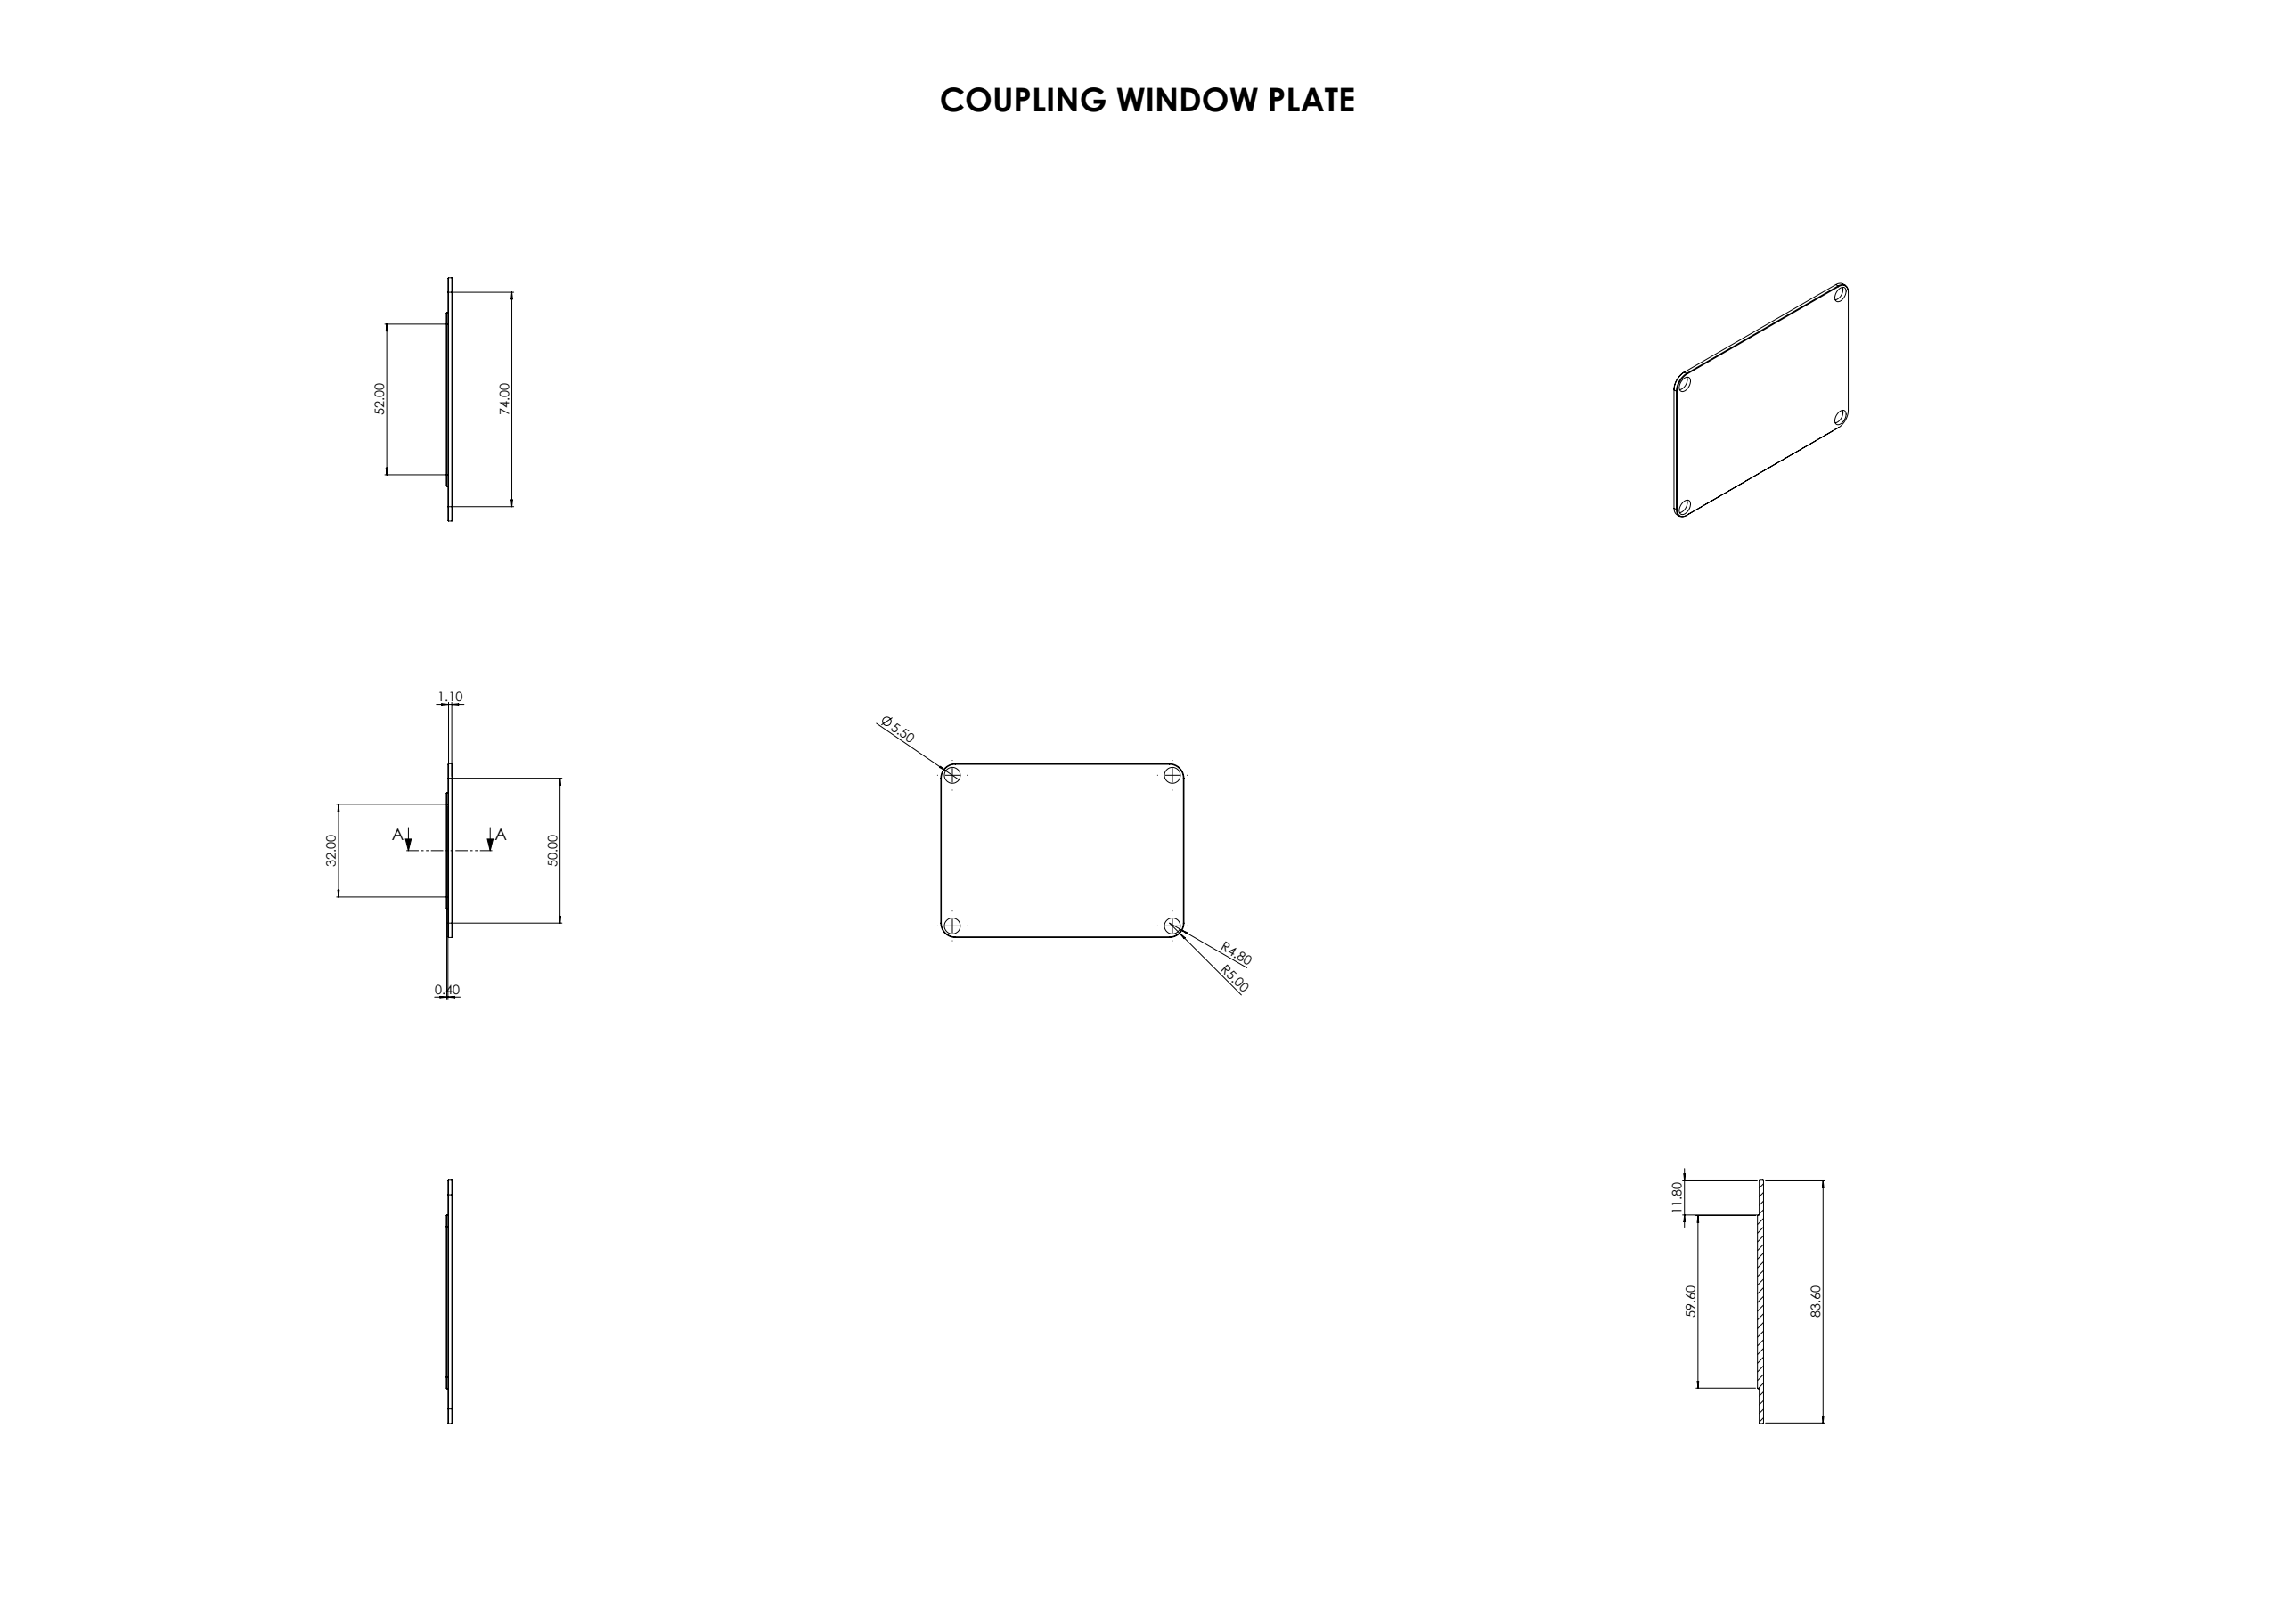
ISO-10303-21;
HEADER;
/* Generated by software containing ST-Developer
 * from STEP Tools, Inc. (www.steptools.com) 
 */

FILE_DESCRIPTION(
/* description */ (''),
/* implementation_level */ '2;1');

FILE_NAME(
/* name */ '18_Coupling_Window_Plate.step',
/* time_stamp */ '2026-10-26T04:15:57-07:00',
/* author */ (''),
/* organization */ (''),
/* preprocessor_version */ 'ST-DEVELOPER v20.2',
/* originating_system */ 'Autodesk Translation Framework v15.15.0.0',
/* authorisation */ '');

FILE_SCHEMA (('AUTOMOTIVE_DESIGN { 1 0 10303 214 3 1 1 }'));
ENDSEC;

DATA;
#10=MECHANICAL_DESIGN_GEOMETRIC_PRESENTATION_REPRESENTATION('',(#466),#55737);
#386=CONICAL_SURFACE('',#29308,4.90000000000002,0.785398163397446);
#387=CONICAL_SURFACE('',#29312,4.90000000000001,0.785398163397446);
#388=CONICAL_SURFACE('',#29316,4.90000000000003,0.785398163397493);
#389=CONICAL_SURFACE('',#29320,4.9,0.785398163397493);
#390=CONICAL_SURFACE('',#29339,4.9,0.785398163397493);
#391=CONICAL_SURFACE('',#29343,4.90000000000003,0.785398163397493);
#392=CONICAL_SURFACE('',#29347,4.90000000000001,0.785398163397446);
#393=CONICAL_SURFACE('',#29350,4.90000000000002,0.785398163397446);
#394=CONICAL_SURFACE('',#29361,3.90000000000002,0.785398163397454);
#395=CONICAL_SURFACE('',#29365,3.90000000000002,0.785398163397446);
#396=CONICAL_SURFACE('',#29369,3.89999999999998,0.785398163397493);
#397=CONICAL_SURFACE('',#29373,3.89999999999997,0.785398163397493);
#426=SHAPE_REPRESENTATION_RELATIONSHIP('SRR','None',#55835,#446);
#446=ADVANCED_BREP_SHAPE_REPRESENTATION('',(#486),#55731);
#466=STYLED_ITEM('',(#55977),#486);
#486=MANIFOLD_SOLID_BREP('Body1',#27235);
#704=FACE_BOUND('',#9610,.T.);
#705=FACE_BOUND('',#9611,.T.);
#706=FACE_BOUND('',#9612,.T.);
#707=FACE_BOUND('',#9613,.T.);
#708=FACE_BOUND('',#9614,.T.);
#709=FACE_BOUND('',#9627,.T.);
#710=FACE_BOUND('',#9628,.T.);
#711=FACE_BOUND('',#9629,.T.);
#712=FACE_BOUND('',#9630,.T.);
#1451=PLANE('',#29307);
#1452=PLANE('',#29311);
#1453=PLANE('',#29315);
#1454=PLANE('',#29319);
#1455=PLANE('',#29325);
#1456=PLANE('',#29328);
#1457=PLANE('',#29329);
#1458=PLANE('',#29338);
#1459=PLANE('',#29342);
#1460=PLANE('',#29346);
#1461=PLANE('',#29349);
#1462=PLANE('',#29353);
#1463=PLANE('',#29355);
#1464=PLANE('',#29360);
#1465=PLANE('',#29364);
#1466=PLANE('',#29368);
#1467=PLANE('',#29372);
#1468=PLANE('',#29377);
#1469=PLANE('',#29379);
#1470=PLANE('',#29380);
#1471=PLANE('',#29382);
#1472=PLANE('',#29384);
#1473=PLANE('',#29389);
#3420=LINE('',#45873,#5791);
#3421=LINE('',#45875,#5792);
#3422=LINE('',#45877,#5793);
#3423=LINE('',#45878,#5794);
#3424=LINE('',#45882,#5795);
#3425=LINE('',#45888,#5796);
#3426=LINE('',#45889,#5797);
#3427=LINE('',#45890,#5798);
#3428=LINE('',#45894,#5799);
#3429=LINE('',#45900,#5800);
#3430=LINE('',#45901,#5801);
#3431=LINE('',#45902,#5802);
#3432=LINE('',#45906,#5803);
#3433=LINE('',#45912,#5804);
#3434=LINE('',#45913,#5805);
#3435=LINE('',#45914,#5806);
#3436=LINE('',#45920,#5807);
#3437=LINE('',#45923,#5808);
#3438=LINE('',#45926,#5809);
#3439=LINE('',#45927,#5810);
#3440=LINE('',#45930,#5811);
#3441=LINE('',#45934,#5812);
#3442=LINE('',#45935,#5813);
#3443=LINE('',#45947,#5814);
#3444=LINE('',#45951,#5815);
#3445=LINE('',#45955,#5816);
#3446=LINE('',#45959,#5817);
#3447=LINE('',#45963,#5818);
#3448=LINE('',#45965,#5819);
#3449=LINE('',#45966,#5820);
#3450=LINE('',#45970,#5821);
#3451=LINE('',#45976,#5822);
#3452=LINE('',#45977,#5823);
#3453=LINE('',#45978,#5824);
#3454=LINE('',#45982,#5825);
#3455=LINE('',#45987,#5826);
#3456=LINE('',#45988,#5827);
#3457=LINE('',#45989,#5828);
#3458=LINE('',#45992,#5829);
#3459=LINE('',#45996,#5830);
#3460=LINE('',#45997,#5831);
#3461=LINE('',#46001,#5832);
#3462=LINE('',#46002,#5833);
#3463=LINE('',#46004,#5834);
#3464=LINE('',#46018,#5835);
#3465=LINE('',#46020,#5836);
#3466=LINE('',#46022,#5837);
#3467=LINE('',#46023,#5838);
#3468=LINE('',#46027,#5839);
#3469=LINE('',#46033,#5840);
#3470=LINE('',#46034,#5841);
#3471=LINE('',#46035,#5842);
#3472=LINE('',#46039,#5843);
#3473=LINE('',#46045,#5844);
#3474=LINE('',#46046,#5845);
#3475=LINE('',#46047,#5846);
#3476=LINE('',#46051,#5847);
#3477=LINE('',#46057,#5848);
#3478=LINE('',#46058,#5849);
#3479=LINE('',#46059,#5850);
#3480=LINE('',#46064,#5851);
#3481=LINE('',#46065,#5852);
#3482=LINE('',#46067,#5853);
#3483=LINE('',#46069,#5854);
#3484=LINE('',#46071,#5855);
#3485=LINE('',#46074,#5856);
#3486=LINE('',#46076,#5857);
#3487=LINE('',#46078,#5858);
#3488=LINE('',#46081,#5859);
#3489=LINE('',#46083,#5860);
#3490=LINE('',#46085,#5861);
#3491=LINE('',#46087,#5862);
#5791=VECTOR('',#35330,10.);
#5792=VECTOR('',#35331,10.);
#5793=VECTOR('',#35332,10.);
#5794=VECTOR('',#35333,10.);
#5795=VECTOR('',#35336,10.);
#5796=VECTOR('',#35343,10.);
#5797=VECTOR('',#35344,10.);
#5798=VECTOR('',#35345,10.);
#5799=VECTOR('',#35348,10.);
#5800=VECTOR('',#35355,10.);
#5801=VECTOR('',#35356,10.);
#5802=VECTOR('',#35357,10.);
#5803=VECTOR('',#35360,10.);
#5804=VECTOR('',#35367,10.);
#5805=VECTOR('',#35368,10.);
#5806=VECTOR('',#35369,10.);
#5807=VECTOR('',#35378,10.);
#5808=VECTOR('',#35381,10.);
#5809=VECTOR('',#35384,10.);
#5810=VECTOR('',#35385,10.);
#5811=VECTOR('',#35388,10.);
#5812=VECTOR('',#35393,10.);
#5813=VECTOR('',#35394,10.);
#5814=VECTOR('',#35405,10.);
#5815=VECTOR('',#35408,10.);
#5816=VECTOR('',#35411,10.);
#5817=VECTOR('',#35414,10.);
#5818=VECTOR('',#35419,10.);
#5819=VECTOR('',#35420,10.);
#5820=VECTOR('',#35421,10.);
#5821=VECTOR('',#35424,10.);
#5822=VECTOR('',#35431,10.);
#5823=VECTOR('',#35432,10.);
#5824=VECTOR('',#35433,10.);
#5825=VECTOR('',#35436,10.);
#5826=VECTOR('',#35443,10.);
#5827=VECTOR('',#35444,10.);
#5828=VECTOR('',#35445,10.);
#5829=VECTOR('',#35448,10.);
#5830=VECTOR('',#35453,10.);
#5831=VECTOR('',#35454,10.);
#5832=VECTOR('',#35461,10.);
#5833=VECTOR('',#35462,10.);
#5834=VECTOR('',#35465,10.);
#5835=VECTOR('',#35480,10.);
#5836=VECTOR('',#35481,10.);
#5837=VECTOR('',#35482,10.);
#5838=VECTOR('',#35483,10.);
#5839=VECTOR('',#35486,10.);
#5840=VECTOR('',#35493,10.);
#5841=VECTOR('',#35494,10.);
#5842=VECTOR('',#35495,10.);
#5843=VECTOR('',#35498,10.);
#5844=VECTOR('',#35505,10.);
#5845=VECTOR('',#35506,10.);
#5846=VECTOR('',#35507,10.);
#5847=VECTOR('',#35510,10.);
#5848=VECTOR('',#35517,10.);
#5849=VECTOR('',#35518,10.);
#5850=VECTOR('',#35519,10.);
#5851=VECTOR('',#35528,10.);
#5852=VECTOR('',#35529,10.);
#5853=VECTOR('',#35532,10.);
#5854=VECTOR('',#35535,10.);
#5855=VECTOR('',#35538,10.);
#5856=VECTOR('',#35543,10.);
#5857=VECTOR('',#35546,10.);
#5858=VECTOR('',#35549,10.);
#5859=VECTOR('',#35554,2.75);
#5860=VECTOR('',#35557,2.75);
#5861=VECTOR('',#35560,2.75);
#5862=VECTOR('',#35563,2.75);
#6699=CYLINDRICAL_SURFACE('',#29323,5.00000000000001);
#6700=CYLINDRICAL_SURFACE('',#29326,5.00000000000002);
#6701=CYLINDRICAL_SURFACE('',#29352,5.00000000000004);
#6702=CYLINDRICAL_SURFACE('',#29354,5.00000000000001);
#6703=CYLINDRICAL_SURFACE('',#29376,4.00000000000002);
#6704=CYLINDRICAL_SURFACE('',#29378,4.00000000000002);
#6705=CYLINDRICAL_SURFACE('',#29381,3.99999999999998);
#6706=CYLINDRICAL_SURFACE('',#29383,3.99999999999999);
#6707=CYLINDRICAL_SURFACE('',#29385,2.75);
#6708=CYLINDRICAL_SURFACE('',#29386,2.75);
#6709=CYLINDRICAL_SURFACE('',#29387,2.75);
#6710=CYLINDRICAL_SURFACE('',#29388,2.75);
#7928=FACE_OUTER_BOUND('',#9597,.T.);
#7929=FACE_OUTER_BOUND('',#9598,.T.);
#7930=FACE_OUTER_BOUND('',#9599,.T.);
#7931=FACE_OUTER_BOUND('',#9600,.T.);
#7932=FACE_OUTER_BOUND('',#9601,.T.);
#7933=FACE_OUTER_BOUND('',#9602,.T.);
#7934=FACE_OUTER_BOUND('',#9603,.T.);
#7935=FACE_OUTER_BOUND('',#9604,.T.);
#7936=FACE_OUTER_BOUND('',#9605,.T.);
#7937=FACE_OUTER_BOUND('',#9606,.T.);
#7938=FACE_OUTER_BOUND('',#9607,.T.);
#7939=FACE_OUTER_BOUND('',#9608,.T.);
#7940=FACE_OUTER_BOUND('',#9609,.T.);
#7941=FACE_OUTER_BOUND('',#9615,.T.);
#7942=FACE_OUTER_BOUND('',#9616,.T.);
#7943=FACE_OUTER_BOUND('',#9617,.T.);
#7944=FACE_OUTER_BOUND('',#9618,.T.);
#7945=FACE_OUTER_BOUND('',#9619,.T.);
#7946=FACE_OUTER_BOUND('',#9620,.T.);
#7947=FACE_OUTER_BOUND('',#9621,.T.);
#7948=FACE_OUTER_BOUND('',#9622,.T.);
#7949=FACE_OUTER_BOUND('',#9623,.T.);
#7950=FACE_OUTER_BOUND('',#9624,.T.);
#7951=FACE_OUTER_BOUND('',#9625,.T.);
#7952=FACE_OUTER_BOUND('',#9626,.T.);
#7953=FACE_OUTER_BOUND('',#9631,.T.);
#7954=FACE_OUTER_BOUND('',#9632,.T.);
#7955=FACE_OUTER_BOUND('',#9633,.T.);
#7956=FACE_OUTER_BOUND('',#9634,.T.);
#7957=FACE_OUTER_BOUND('',#9635,.T.);
#7958=FACE_OUTER_BOUND('',#9636,.T.);
#7959=FACE_OUTER_BOUND('',#9637,.T.);
#7960=FACE_OUTER_BOUND('',#9638,.T.);
#7961=FACE_OUTER_BOUND('',#9639,.T.);
#7962=FACE_OUTER_BOUND('',#9640,.T.);
#7963=FACE_OUTER_BOUND('',#9641,.T.);
#7964=FACE_OUTER_BOUND('',#9642,.T.);
#7965=FACE_OUTER_BOUND('',#9643,.T.);
#7966=FACE_OUTER_BOUND('',#9644,.T.);
#7967=FACE_OUTER_BOUND('',#9645,.T.);
#7968=FACE_OUTER_BOUND('',#9646,.T.);
#7969=FACE_OUTER_BOUND('',#9647,.T.);
#7970=FACE_OUTER_BOUND('',#9648,.T.);
#7971=FACE_OUTER_BOUND('',#9649,.T.);
#7972=FACE_OUTER_BOUND('',#9650,.T.);
#7973=FACE_OUTER_BOUND('',#9651,.T.);
#7974=FACE_OUTER_BOUND('',#9652,.T.);
#9597=EDGE_LOOP('',(#23306,#23307,#23308,#23309));
#9598=EDGE_LOOP('',(#23310,#23311,#23312,#23313));
#9599=EDGE_LOOP('',(#23314,#23315,#23316,#23317));
#9600=EDGE_LOOP('',(#23318,#23319,#23320,#23321));
#9601=EDGE_LOOP('',(#23322,#23323,#23324,#23325));
#9602=EDGE_LOOP('',(#23326,#23327,#23328,#23329));
#9603=EDGE_LOOP('',(#23330,#23331,#23332,#23333));
#9604=EDGE_LOOP('',(#23334,#23335,#23336,#23337));
#9605=EDGE_LOOP('',(#23338,#23339,#23340,#23341));
#9606=EDGE_LOOP('',(#23342,#23343,#23344,#23345));
#9607=EDGE_LOOP('',(#23346,#23347,#23348,#23349));
#9608=EDGE_LOOP('',(#23350,#23351,#23352,#23353));
#9609=EDGE_LOOP('',(#23354,#23355,#23356,#23357,#23358,#23359,#23360,#23361));
#9610=EDGE_LOOP('',(#23362));
#9611=EDGE_LOOP('',(#23363));
#9612=EDGE_LOOP('',(#23364));
#9613=EDGE_LOOP('',(#23365));
#9614=EDGE_LOOP('',(#23366,#23367,#23368,#23369,#23370,#23371,#23372,#23373));
#9615=EDGE_LOOP('',(#23374,#23375,#23376,#23377));
#9616=EDGE_LOOP('',(#23378,#23379,#23380,#23381));
#9617=EDGE_LOOP('',(#23382,#23383,#23384,#23385));
#9618=EDGE_LOOP('',(#23386,#23387,#23388,#23389));
#9619=EDGE_LOOP('',(#23390,#23391,#23392,#23393));
#9620=EDGE_LOOP('',(#23394,#23395,#23396,#23397));
#9621=EDGE_LOOP('',(#23398,#23399,#23400,#23401));
#9622=EDGE_LOOP('',(#23402,#23403,#23404,#23405));
#9623=EDGE_LOOP('',(#23406,#23407,#23408,#23409));
#9624=EDGE_LOOP('',(#23410,#23411,#23412,#23413));
#9625=EDGE_LOOP('',(#23414,#23415,#23416,#23417));
#9626=EDGE_LOOP('',(#23418,#23419,#23420,#23421,#23422,#23423,#23424,#23425));
#9627=EDGE_LOOP('',(#23426));
#9628=EDGE_LOOP('',(#23427));
#9629=EDGE_LOOP('',(#23428));
#9630=EDGE_LOOP('',(#23429));
#9631=EDGE_LOOP('',(#23430,#23431,#23432,#23433));
#9632=EDGE_LOOP('',(#23434,#23435,#23436,#23437));
#9633=EDGE_LOOP('',(#23438,#23439,#23440,#23441));
#9634=EDGE_LOOP('',(#23442,#23443,#23444,#23445));
#9635=EDGE_LOOP('',(#23446,#23447,#23448,#23449));
#9636=EDGE_LOOP('',(#23450,#23451,#23452,#23453));
#9637=EDGE_LOOP('',(#23454,#23455,#23456,#23457));
#9638=EDGE_LOOP('',(#23458,#23459,#23460,#23461));
#9639=EDGE_LOOP('',(#23462,#23463,#23464,#23465));
#9640=EDGE_LOOP('',(#23466,#23467,#23468,#23469));
#9641=EDGE_LOOP('',(#23470,#23471,#23472,#23473));
#9642=EDGE_LOOP('',(#23474,#23475,#23476,#23477));
#9643=EDGE_LOOP('',(#23478,#23479,#23480,#23481,#23482,#23483,#23484,#23485));
#9644=EDGE_LOOP('',(#23486,#23487,#23488,#23489));
#9645=EDGE_LOOP('',(#23490,#23491,#23492,#23493));
#9646=EDGE_LOOP('',(#23494,#23495,#23496,#23497));
#9647=EDGE_LOOP('',(#23498,#23499,#23500,#23501));
#9648=EDGE_LOOP('',(#23502,#23503,#23504,#23505));
#9649=EDGE_LOOP('',(#23506,#23507,#23508,#23509));
#9650=EDGE_LOOP('',(#23510,#23511,#23512,#23513));
#9651=EDGE_LOOP('',(#23514,#23515,#23516,#23517));
#9652=EDGE_LOOP('',(#23518,#23519,#23520,#23521));
#10811=CIRCLE('',#29309,4.80000000000002);
#10812=CIRCLE('',#29310,5.00000000000002);
#10813=CIRCLE('',#29313,4.80000000000001);
#10814=CIRCLE('',#29314,5.00000000000001);
#10815=CIRCLE('',#29317,4.80000000000002);
#10816=CIRCLE('',#29318,5.00000000000004);
#10817=CIRCLE('',#29321,4.8);
#10818=CIRCLE('',#29322,5.00000000000001);
#10819=CIRCLE('',#29324,5.00000000000001);
#10820=CIRCLE('',#29327,5.00000000000002);
#10821=CIRCLE('',#29330,2.75);
#10822=CIRCLE('',#29331,2.75);
#10823=CIRCLE('',#29332,2.75);
#10824=CIRCLE('',#29333,2.75);
#10825=CIRCLE('',#29334,3.99999999999998);
#10826=CIRCLE('',#29335,3.99999999999999);
#10827=CIRCLE('',#29336,4.00000000000002);
#10828=CIRCLE('',#29337,4.00000000000002);
#10829=CIRCLE('',#29340,4.8);
#10830=CIRCLE('',#29341,5.00000000000001);
#10831=CIRCLE('',#29344,4.80000000000002);
#10832=CIRCLE('',#29345,5.00000000000004);
#10833=CIRCLE('',#29348,4.80000000000001);
#10834=CIRCLE('',#29351,4.80000000000002);
#10835=CIRCLE('',#29356,2.75);
#10836=CIRCLE('',#29357,2.75);
#10837=CIRCLE('',#29358,2.75);
#10838=CIRCLE('',#29359,2.75);
#10839=CIRCLE('',#29362,3.80000000000002);
#10840=CIRCLE('',#29363,4.00000000000002);
#10841=CIRCLE('',#29366,3.80000000000002);
#10842=CIRCLE('',#29367,4.00000000000002);
#10843=CIRCLE('',#29370,3.79999999999997);
#10844=CIRCLE('',#29371,3.99999999999999);
#10845=CIRCLE('',#29374,3.79999999999997);
#10846=CIRCLE('',#29375,3.99999999999998);
#13176=VERTEX_POINT('',#45871);
#13177=VERTEX_POINT('',#45872);
#13178=VERTEX_POINT('',#45874);
#13179=VERTEX_POINT('',#45876);
#13180=VERTEX_POINT('',#45880);
#13181=VERTEX_POINT('',#45881);
#13182=VERTEX_POINT('',#45886);
#13183=VERTEX_POINT('',#45887);
#13184=VERTEX_POINT('',#45892);
#13185=VERTEX_POINT('',#45893);
#13186=VERTEX_POINT('',#45898);
#13187=VERTEX_POINT('',#45899);
#13188=VERTEX_POINT('',#45904);
#13189=VERTEX_POINT('',#45905);
#13190=VERTEX_POINT('',#45910);
#13191=VERTEX_POINT('',#45911);
#13192=VERTEX_POINT('',#45919);
#13193=VERTEX_POINT('',#45921);
#13194=VERTEX_POINT('',#45925);
#13195=VERTEX_POINT('',#45929);
#13196=VERTEX_POINT('',#45933);
#13197=VERTEX_POINT('',#45937);
#13198=VERTEX_POINT('',#45939);
#13199=VERTEX_POINT('',#45941);
#13200=VERTEX_POINT('',#45943);
#13201=VERTEX_POINT('',#45945);
#13202=VERTEX_POINT('',#45946);
#13203=VERTEX_POINT('',#45948);
#13204=VERTEX_POINT('',#45950);
#13205=VERTEX_POINT('',#45952);
#13206=VERTEX_POINT('',#45954);
#13207=VERTEX_POINT('',#45956);
#13208=VERTEX_POINT('',#45958);
#13209=VERTEX_POINT('',#45962);
#13210=VERTEX_POINT('',#45964);
#13211=VERTEX_POINT('',#45968);
#13212=VERTEX_POINT('',#45969);
#13213=VERTEX_POINT('',#45974);
#13214=VERTEX_POINT('',#45975);
#13215=VERTEX_POINT('',#45980);
#13216=VERTEX_POINT('',#45981);
#13217=VERTEX_POINT('',#45986);
#13218=VERTEX_POINT('',#45991);
#13219=VERTEX_POINT('',#45995);
#13220=VERTEX_POINT('',#46007);
#13221=VERTEX_POINT('',#46009);
#13222=VERTEX_POINT('',#46011);
#13223=VERTEX_POINT('',#46013);
#13224=VERTEX_POINT('',#46016);
#13225=VERTEX_POINT('',#46017);
#13226=VERTEX_POINT('',#46019);
#13227=VERTEX_POINT('',#46021);
#13228=VERTEX_POINT('',#46025);
#13229=VERTEX_POINT('',#46026);
#13230=VERTEX_POINT('',#46031);
#13231=VERTEX_POINT('',#46032);
#13232=VERTEX_POINT('',#46037);
#13233=VERTEX_POINT('',#46038);
#13234=VERTEX_POINT('',#46043);
#13235=VERTEX_POINT('',#46044);
#13236=VERTEX_POINT('',#46049);
#13237=VERTEX_POINT('',#46050);
#13238=VERTEX_POINT('',#46055);
#13239=VERTEX_POINT('',#46056);
#16657=EDGE_CURVE('',#13176,#13177,#3420,.T.);
#16658=EDGE_CURVE('',#13177,#13178,#3421,.T.);
#16659=EDGE_CURVE('',#13178,#13179,#3422,.T.);
#16660=EDGE_CURVE('',#13179,#13176,#3423,.T.);
#16661=EDGE_CURVE('',#13180,#13181,#3424,.T.);
#16662=EDGE_CURVE('',#13181,#13177,#10811,.T.);
#16663=EDGE_CURVE('',#13176,#13180,#10812,.T.);
#16664=EDGE_CURVE('',#13182,#13183,#3425,.T.);
#16665=EDGE_CURVE('',#13183,#13181,#3426,.T.);
#16666=EDGE_CURVE('',#13180,#13182,#3427,.T.);
#16667=EDGE_CURVE('',#13184,#13185,#3428,.T.);
#16668=EDGE_CURVE('',#13185,#13183,#10813,.T.);
#16669=EDGE_CURVE('',#13182,#13184,#10814,.T.);
#16670=EDGE_CURVE('',#13186,#13187,#3429,.T.);
#16671=EDGE_CURVE('',#13187,#13185,#3430,.T.);
#16672=EDGE_CURVE('',#13184,#13186,#3431,.T.);
#16673=EDGE_CURVE('',#13188,#13189,#3432,.T.);
#16674=EDGE_CURVE('',#13189,#13187,#10815,.T.);
#16675=EDGE_CURVE('',#13186,#13188,#10816,.T.);
#16676=EDGE_CURVE('',#13190,#13191,#3433,.T.);
#16677=EDGE_CURVE('',#13191,#13189,#3434,.T.);
#16678=EDGE_CURVE('',#13188,#13190,#3435,.T.);
#16679=EDGE_CURVE('',#13178,#13191,#10817,.T.);
#16680=EDGE_CURVE('',#13190,#13179,#10818,.T.);
#16681=EDGE_CURVE('',#13192,#13182,#3436,.T.);
#16682=EDGE_CURVE('',#13193,#13192,#10819,.T.);
#16683=EDGE_CURVE('',#13193,#13184,#3437,.T.);
#16684=EDGE_CURVE('',#13194,#13180,#3438,.T.);
#16685=EDGE_CURVE('',#13192,#13194,#3439,.T.);
#16686=EDGE_CURVE('',#13195,#13176,#3440,.T.);
#16687=EDGE_CURVE('',#13194,#13195,#10820,.T.);
#16688=EDGE_CURVE('',#13196,#13179,#3441,.T.);
#16689=EDGE_CURVE('',#13195,#13196,#3442,.T.);
#16690=EDGE_CURVE('',#13197,#13197,#10821,.T.);
#16691=EDGE_CURVE('',#13198,#13198,#10822,.T.);
#16692=EDGE_CURVE('',#13199,#13199,#10823,.T.);
#16693=EDGE_CURVE('',#13200,#13200,#10824,.T.);
#16694=EDGE_CURVE('',#13201,#13202,#3443,.T.);
#16695=EDGE_CURVE('',#13202,#13203,#10825,.T.);
#16696=EDGE_CURVE('',#13203,#13204,#3444,.T.);
#16697=EDGE_CURVE('',#13204,#13205,#10826,.T.);
#16698=EDGE_CURVE('',#13205,#13206,#3445,.T.);
#16699=EDGE_CURVE('',#13206,#13207,#10827,.T.);
#16700=EDGE_CURVE('',#13207,#13208,#3446,.T.);
#16701=EDGE_CURVE('',#13208,#13201,#10828,.T.);
#16702=EDGE_CURVE('',#13196,#13209,#3447,.T.);
#16703=EDGE_CURVE('',#13209,#13210,#3448,.T.);
#16704=EDGE_CURVE('',#13210,#13195,#3449,.T.);
#16705=EDGE_CURVE('',#13211,#13212,#3450,.T.);
#16706=EDGE_CURVE('',#13212,#13209,#10829,.T.);
#16707=EDGE_CURVE('',#13196,#13211,#10830,.T.);
#16708=EDGE_CURVE('',#13213,#13214,#3451,.T.);
#16709=EDGE_CURVE('',#13214,#13212,#3452,.T.);
#16710=EDGE_CURVE('',#13211,#13213,#3453,.T.);
#16711=EDGE_CURVE('',#13215,#13216,#3454,.T.);
#16712=EDGE_CURVE('',#13216,#13214,#10831,.T.);
#16713=EDGE_CURVE('',#13213,#13215,#10832,.T.);
#16714=EDGE_CURVE('',#13193,#13217,#3455,.T.);
#16715=EDGE_CURVE('',#13217,#13216,#3456,.T.);
#16716=EDGE_CURVE('',#13215,#13193,#3457,.T.);
#16717=EDGE_CURVE('',#13192,#13218,#3458,.T.);
#16718=EDGE_CURVE('',#13218,#13217,#10833,.T.);
#16719=EDGE_CURVE('',#13194,#13219,#3459,.T.);
#16720=EDGE_CURVE('',#13219,#13218,#3460,.T.);
#16721=EDGE_CURVE('',#13210,#13219,#10834,.T.);
#16722=EDGE_CURVE('',#13215,#13186,#3461,.T.);
#16723=EDGE_CURVE('',#13213,#13188,#3462,.T.);
#16724=EDGE_CURVE('',#13211,#13190,#3463,.T.);
#16725=EDGE_CURVE('',#13220,#13220,#10835,.T.);
#16726=EDGE_CURVE('',#13221,#13221,#10836,.T.);
#16727=EDGE_CURVE('',#13222,#13222,#10837,.T.);
#16728=EDGE_CURVE('',#13223,#13223,#10838,.T.);
#16729=EDGE_CURVE('',#13224,#13225,#3464,.T.);
#16730=EDGE_CURVE('',#13225,#13226,#3465,.T.);
#16731=EDGE_CURVE('',#13226,#13227,#3466,.T.);
#16732=EDGE_CURVE('',#13227,#13224,#3467,.T.);
#16733=EDGE_CURVE('',#13228,#13229,#3468,.T.);
#16734=EDGE_CURVE('',#13229,#13225,#10839,.T.);
#16735=EDGE_CURVE('',#13224,#13228,#10840,.T.);
#16736=EDGE_CURVE('',#13230,#13231,#3469,.T.);
#16737=EDGE_CURVE('',#13231,#13229,#3470,.T.);
#16738=EDGE_CURVE('',#13228,#13230,#3471,.T.);
#16739=EDGE_CURVE('',#13232,#13233,#3472,.T.);
#16740=EDGE_CURVE('',#13233,#13231,#10841,.T.);
#16741=EDGE_CURVE('',#13230,#13232,#10842,.T.);
#16742=EDGE_CURVE('',#13234,#13235,#3473,.T.);
#16743=EDGE_CURVE('',#13235,#13233,#3474,.T.);
#16744=EDGE_CURVE('',#13232,#13234,#3475,.T.);
#16745=EDGE_CURVE('',#13236,#13237,#3476,.T.);
#16746=EDGE_CURVE('',#13237,#13235,#10843,.T.);
#16747=EDGE_CURVE('',#13234,#13236,#10844,.T.);
#16748=EDGE_CURVE('',#13238,#13239,#3477,.T.);
#16749=EDGE_CURVE('',#13239,#13237,#3478,.T.);
#16750=EDGE_CURVE('',#13236,#13238,#3479,.T.);
#16751=EDGE_CURVE('',#13226,#13239,#10845,.T.);
#16752=EDGE_CURVE('',#13238,#13227,#10846,.T.);
#16753=EDGE_CURVE('',#13207,#13230,#3480,.T.);
#16754=EDGE_CURVE('',#13206,#13232,#3481,.T.);
#16755=EDGE_CURVE('',#13208,#13228,#3482,.T.);
#16756=EDGE_CURVE('',#13201,#13224,#3483,.T.);
#16757=EDGE_CURVE('',#13202,#13227,#3484,.T.);
#16758=EDGE_CURVE('',#13203,#13238,#3485,.T.);
#16759=EDGE_CURVE('',#13204,#13236,#3486,.T.);
#16760=EDGE_CURVE('',#13205,#13234,#3487,.T.);
#16761=EDGE_CURVE('',#13223,#13200,#3488,.T.);
#16762=EDGE_CURVE('',#13222,#13199,#3489,.T.);
#16763=EDGE_CURVE('',#13221,#13198,#3490,.T.);
#16764=EDGE_CURVE('',#13220,#13197,#3491,.T.);
#23306=ORIENTED_EDGE('',*,*,#16657,.T.);
#23307=ORIENTED_EDGE('',*,*,#16658,.T.);
#23308=ORIENTED_EDGE('',*,*,#16659,.T.);
#23309=ORIENTED_EDGE('',*,*,#16660,.T.);
#23310=ORIENTED_EDGE('',*,*,#16661,.T.);
#23311=ORIENTED_EDGE('',*,*,#16662,.T.);
#23312=ORIENTED_EDGE('',*,*,#16657,.F.);
#23313=ORIENTED_EDGE('',*,*,#16663,.T.);
#23314=ORIENTED_EDGE('',*,*,#16664,.T.);
#23315=ORIENTED_EDGE('',*,*,#16665,.T.);
#23316=ORIENTED_EDGE('',*,*,#16661,.F.);
#23317=ORIENTED_EDGE('',*,*,#16666,.T.);
#23318=ORIENTED_EDGE('',*,*,#16667,.T.);
#23319=ORIENTED_EDGE('',*,*,#16668,.T.);
#23320=ORIENTED_EDGE('',*,*,#16664,.F.);
#23321=ORIENTED_EDGE('',*,*,#16669,.T.);
#23322=ORIENTED_EDGE('',*,*,#16670,.T.);
#23323=ORIENTED_EDGE('',*,*,#16671,.T.);
#23324=ORIENTED_EDGE('',*,*,#16667,.F.);
#23325=ORIENTED_EDGE('',*,*,#16672,.T.);
#23326=ORIENTED_EDGE('',*,*,#16673,.T.);
#23327=ORIENTED_EDGE('',*,*,#16674,.T.);
#23328=ORIENTED_EDGE('',*,*,#16670,.F.);
#23329=ORIENTED_EDGE('',*,*,#16675,.T.);
#23330=ORIENTED_EDGE('',*,*,#16676,.T.);
#23331=ORIENTED_EDGE('',*,*,#16677,.T.);
#23332=ORIENTED_EDGE('',*,*,#16673,.F.);
#23333=ORIENTED_EDGE('',*,*,#16678,.T.);
#23334=ORIENTED_EDGE('',*,*,#16659,.F.);
#23335=ORIENTED_EDGE('',*,*,#16679,.T.);
#23336=ORIENTED_EDGE('',*,*,#16676,.F.);
#23337=ORIENTED_EDGE('',*,*,#16680,.T.);
#23338=ORIENTED_EDGE('',*,*,#16669,.F.);
#23339=ORIENTED_EDGE('',*,*,#16681,.F.);
#23340=ORIENTED_EDGE('',*,*,#16682,.F.);
#23341=ORIENTED_EDGE('',*,*,#16683,.T.);
#23342=ORIENTED_EDGE('',*,*,#16666,.F.);
#23343=ORIENTED_EDGE('',*,*,#16684,.F.);
#23344=ORIENTED_EDGE('',*,*,#16685,.F.);
#23345=ORIENTED_EDGE('',*,*,#16681,.T.);
#23346=ORIENTED_EDGE('',*,*,#16663,.F.);
#23347=ORIENTED_EDGE('',*,*,#16686,.F.);
#23348=ORIENTED_EDGE('',*,*,#16687,.F.);
#23349=ORIENTED_EDGE('',*,*,#16684,.T.);
#23350=ORIENTED_EDGE('',*,*,#16660,.F.);
#23351=ORIENTED_EDGE('',*,*,#16688,.F.);
#23352=ORIENTED_EDGE('',*,*,#16689,.F.);
#23353=ORIENTED_EDGE('',*,*,#16686,.T.);
#23354=ORIENTED_EDGE('',*,*,#16658,.F.);
#23355=ORIENTED_EDGE('',*,*,#16662,.F.);
#23356=ORIENTED_EDGE('',*,*,#16665,.F.);
#23357=ORIENTED_EDGE('',*,*,#16668,.F.);
#23358=ORIENTED_EDGE('',*,*,#16671,.F.);
#23359=ORIENTED_EDGE('',*,*,#16674,.F.);
#23360=ORIENTED_EDGE('',*,*,#16677,.F.);
#23361=ORIENTED_EDGE('',*,*,#16679,.F.);
#23362=ORIENTED_EDGE('',*,*,#16690,.T.);
#23363=ORIENTED_EDGE('',*,*,#16691,.T.);
#23364=ORIENTED_EDGE('',*,*,#16692,.T.);
#23365=ORIENTED_EDGE('',*,*,#16693,.T.);
#23366=ORIENTED_EDGE('',*,*,#16694,.T.);
#23367=ORIENTED_EDGE('',*,*,#16695,.T.);
#23368=ORIENTED_EDGE('',*,*,#16696,.T.);
#23369=ORIENTED_EDGE('',*,*,#16697,.T.);
#23370=ORIENTED_EDGE('',*,*,#16698,.T.);
#23371=ORIENTED_EDGE('',*,*,#16699,.T.);
#23372=ORIENTED_EDGE('',*,*,#16700,.T.);
#23373=ORIENTED_EDGE('',*,*,#16701,.T.);
#23374=ORIENTED_EDGE('',*,*,#16702,.T.);
#23375=ORIENTED_EDGE('',*,*,#16703,.T.);
#23376=ORIENTED_EDGE('',*,*,#16704,.T.);
#23377=ORIENTED_EDGE('',*,*,#16689,.T.);
#23378=ORIENTED_EDGE('',*,*,#16705,.T.);
#23379=ORIENTED_EDGE('',*,*,#16706,.T.);
#23380=ORIENTED_EDGE('',*,*,#16702,.F.);
#23381=ORIENTED_EDGE('',*,*,#16707,.T.);
#23382=ORIENTED_EDGE('',*,*,#16708,.T.);
#23383=ORIENTED_EDGE('',*,*,#16709,.T.);
#23384=ORIENTED_EDGE('',*,*,#16705,.F.);
#23385=ORIENTED_EDGE('',*,*,#16710,.T.);
#23386=ORIENTED_EDGE('',*,*,#16711,.T.);
#23387=ORIENTED_EDGE('',*,*,#16712,.T.);
#23388=ORIENTED_EDGE('',*,*,#16708,.F.);
#23389=ORIENTED_EDGE('',*,*,#16713,.T.);
#23390=ORIENTED_EDGE('',*,*,#16714,.T.);
#23391=ORIENTED_EDGE('',*,*,#16715,.T.);
#23392=ORIENTED_EDGE('',*,*,#16711,.F.);
#23393=ORIENTED_EDGE('',*,*,#16716,.T.);
#23394=ORIENTED_EDGE('',*,*,#16717,.T.);
#23395=ORIENTED_EDGE('',*,*,#16718,.T.);
#23396=ORIENTED_EDGE('',*,*,#16714,.F.);
#23397=ORIENTED_EDGE('',*,*,#16682,.T.);
#23398=ORIENTED_EDGE('',*,*,#16719,.T.);
#23399=ORIENTED_EDGE('',*,*,#16720,.T.);
#23400=ORIENTED_EDGE('',*,*,#16717,.F.);
#23401=ORIENTED_EDGE('',*,*,#16685,.T.);
#23402=ORIENTED_EDGE('',*,*,#16704,.F.);
#23403=ORIENTED_EDGE('',*,*,#16721,.T.);
#23404=ORIENTED_EDGE('',*,*,#16719,.F.);
#23405=ORIENTED_EDGE('',*,*,#16687,.T.);
#23406=ORIENTED_EDGE('',*,*,#16675,.F.);
#23407=ORIENTED_EDGE('',*,*,#16722,.F.);
#23408=ORIENTED_EDGE('',*,*,#16713,.F.);
#23409=ORIENTED_EDGE('',*,*,#16723,.T.);
#23410=ORIENTED_EDGE('',*,*,#16678,.F.);
#23411=ORIENTED_EDGE('',*,*,#16723,.F.);
#23412=ORIENTED_EDGE('',*,*,#16710,.F.);
#23413=ORIENTED_EDGE('',*,*,#16724,.T.);
#23414=ORIENTED_EDGE('',*,*,#16680,.F.);
#23415=ORIENTED_EDGE('',*,*,#16724,.F.);
#23416=ORIENTED_EDGE('',*,*,#16707,.F.);
#23417=ORIENTED_EDGE('',*,*,#16688,.T.);
#23418=ORIENTED_EDGE('',*,*,#16703,.F.);
#23419=ORIENTED_EDGE('',*,*,#16706,.F.);
#23420=ORIENTED_EDGE('',*,*,#16709,.F.);
#23421=ORIENTED_EDGE('',*,*,#16712,.F.);
#23422=ORIENTED_EDGE('',*,*,#16715,.F.);
#23423=ORIENTED_EDGE('',*,*,#16718,.F.);
#23424=ORIENTED_EDGE('',*,*,#16720,.F.);
#23425=ORIENTED_EDGE('',*,*,#16721,.F.);
#23426=ORIENTED_EDGE('',*,*,#16725,.T.);
#23427=ORIENTED_EDGE('',*,*,#16726,.T.);
#23428=ORIENTED_EDGE('',*,*,#16727,.T.);
#23429=ORIENTED_EDGE('',*,*,#16728,.T.);
#23430=ORIENTED_EDGE('',*,*,#16729,.T.);
#23431=ORIENTED_EDGE('',*,*,#16730,.T.);
#23432=ORIENTED_EDGE('',*,*,#16731,.T.);
#23433=ORIENTED_EDGE('',*,*,#16732,.T.);
#23434=ORIENTED_EDGE('',*,*,#16733,.T.);
#23435=ORIENTED_EDGE('',*,*,#16734,.T.);
#23436=ORIENTED_EDGE('',*,*,#16729,.F.);
#23437=ORIENTED_EDGE('',*,*,#16735,.T.);
#23438=ORIENTED_EDGE('',*,*,#16736,.T.);
#23439=ORIENTED_EDGE('',*,*,#16737,.T.);
#23440=ORIENTED_EDGE('',*,*,#16733,.F.);
#23441=ORIENTED_EDGE('',*,*,#16738,.T.);
#23442=ORIENTED_EDGE('',*,*,#16739,.T.);
#23443=ORIENTED_EDGE('',*,*,#16740,.T.);
#23444=ORIENTED_EDGE('',*,*,#16736,.F.);
#23445=ORIENTED_EDGE('',*,*,#16741,.T.);
#23446=ORIENTED_EDGE('',*,*,#16742,.T.);
#23447=ORIENTED_EDGE('',*,*,#16743,.T.);
#23448=ORIENTED_EDGE('',*,*,#16739,.F.);
#23449=ORIENTED_EDGE('',*,*,#16744,.T.);
#23450=ORIENTED_EDGE('',*,*,#16745,.T.);
#23451=ORIENTED_EDGE('',*,*,#16746,.T.);
#23452=ORIENTED_EDGE('',*,*,#16742,.F.);
#23453=ORIENTED_EDGE('',*,*,#16747,.T.);
#23454=ORIENTED_EDGE('',*,*,#16748,.T.);
#23455=ORIENTED_EDGE('',*,*,#16749,.T.);
#23456=ORIENTED_EDGE('',*,*,#16745,.F.);
#23457=ORIENTED_EDGE('',*,*,#16750,.T.);
#23458=ORIENTED_EDGE('',*,*,#16731,.F.);
#23459=ORIENTED_EDGE('',*,*,#16751,.T.);
#23460=ORIENTED_EDGE('',*,*,#16748,.F.);
#23461=ORIENTED_EDGE('',*,*,#16752,.T.);
#23462=ORIENTED_EDGE('',*,*,#16741,.F.);
#23463=ORIENTED_EDGE('',*,*,#16753,.F.);
#23464=ORIENTED_EDGE('',*,*,#16699,.F.);
#23465=ORIENTED_EDGE('',*,*,#16754,.T.);
#23466=ORIENTED_EDGE('',*,*,#16738,.F.);
#23467=ORIENTED_EDGE('',*,*,#16755,.F.);
#23468=ORIENTED_EDGE('',*,*,#16700,.F.);
#23469=ORIENTED_EDGE('',*,*,#16753,.T.);
#23470=ORIENTED_EDGE('',*,*,#16735,.F.);
#23471=ORIENTED_EDGE('',*,*,#16756,.F.);
#23472=ORIENTED_EDGE('',*,*,#16701,.F.);
#23473=ORIENTED_EDGE('',*,*,#16755,.T.);
#23474=ORIENTED_EDGE('',*,*,#16732,.F.);
#23475=ORIENTED_EDGE('',*,*,#16757,.F.);
#23476=ORIENTED_EDGE('',*,*,#16694,.F.);
#23477=ORIENTED_EDGE('',*,*,#16756,.T.);
#23478=ORIENTED_EDGE('',*,*,#16730,.F.);
#23479=ORIENTED_EDGE('',*,*,#16734,.F.);
#23480=ORIENTED_EDGE('',*,*,#16737,.F.);
#23481=ORIENTED_EDGE('',*,*,#16740,.F.);
#23482=ORIENTED_EDGE('',*,*,#16743,.F.);
#23483=ORIENTED_EDGE('',*,*,#16746,.F.);
#23484=ORIENTED_EDGE('',*,*,#16749,.F.);
#23485=ORIENTED_EDGE('',*,*,#16751,.F.);
#23486=ORIENTED_EDGE('',*,*,#16752,.F.);
#23487=ORIENTED_EDGE('',*,*,#16758,.F.);
#23488=ORIENTED_EDGE('',*,*,#16695,.F.);
#23489=ORIENTED_EDGE('',*,*,#16757,.T.);
#23490=ORIENTED_EDGE('',*,*,#16750,.F.);
#23491=ORIENTED_EDGE('',*,*,#16759,.F.);
#23492=ORIENTED_EDGE('',*,*,#16696,.F.);
#23493=ORIENTED_EDGE('',*,*,#16758,.T.);
#23494=ORIENTED_EDGE('',*,*,#16747,.F.);
#23495=ORIENTED_EDGE('',*,*,#16760,.F.);
#23496=ORIENTED_EDGE('',*,*,#16697,.F.);
#23497=ORIENTED_EDGE('',*,*,#16759,.T.);
#23498=ORIENTED_EDGE('',*,*,#16744,.F.);
#23499=ORIENTED_EDGE('',*,*,#16754,.F.);
#23500=ORIENTED_EDGE('',*,*,#16698,.F.);
#23501=ORIENTED_EDGE('',*,*,#16760,.T.);
#23502=ORIENTED_EDGE('',*,*,#16728,.F.);
#23503=ORIENTED_EDGE('',*,*,#16761,.T.);
#23504=ORIENTED_EDGE('',*,*,#16693,.F.);
#23505=ORIENTED_EDGE('',*,*,#16761,.F.);
#23506=ORIENTED_EDGE('',*,*,#16727,.F.);
#23507=ORIENTED_EDGE('',*,*,#16762,.T.);
#23508=ORIENTED_EDGE('',*,*,#16692,.F.);
#23509=ORIENTED_EDGE('',*,*,#16762,.F.);
#23510=ORIENTED_EDGE('',*,*,#16726,.F.);
#23511=ORIENTED_EDGE('',*,*,#16763,.T.);
#23512=ORIENTED_EDGE('',*,*,#16691,.F.);
#23513=ORIENTED_EDGE('',*,*,#16763,.F.);
#23514=ORIENTED_EDGE('',*,*,#16725,.F.);
#23515=ORIENTED_EDGE('',*,*,#16764,.T.);
#23516=ORIENTED_EDGE('',*,*,#16690,.F.);
#23517=ORIENTED_EDGE('',*,*,#16764,.F.);
#23518=ORIENTED_EDGE('',*,*,#16672,.F.);
#23519=ORIENTED_EDGE('',*,*,#16683,.F.);
#23520=ORIENTED_EDGE('',*,*,#16716,.F.);
#23521=ORIENTED_EDGE('',*,*,#16722,.T.);
#26752=ADVANCED_FACE('',(#7928),#1451,.T.);
#26753=ADVANCED_FACE('',(#7929),#386,.T.);
#26754=ADVANCED_FACE('',(#7930),#1452,.T.);
#26755=ADVANCED_FACE('',(#7931),#387,.T.);
#26756=ADVANCED_FACE('',(#7932),#1453,.T.);
#26757=ADVANCED_FACE('',(#7933),#388,.T.);
#26758=ADVANCED_FACE('',(#7934),#1454,.T.);
#26759=ADVANCED_FACE('',(#7935),#389,.T.);
#26760=ADVANCED_FACE('',(#7936),#6699,.T.);
#26761=ADVANCED_FACE('',(#7937),#1455,.T.);
#26762=ADVANCED_FACE('',(#7938),#6700,.T.);
#26763=ADVANCED_FACE('',(#7939),#1456,.T.);
#26764=ADVANCED_FACE('',(#7940,#704,#705,#706,#707,#708),#1457,.F.);
#26765=ADVANCED_FACE('',(#7941),#1458,.T.);
#26766=ADVANCED_FACE('',(#7942),#390,.T.);
#26767=ADVANCED_FACE('',(#7943),#1459,.T.);
#26768=ADVANCED_FACE('',(#7944),#391,.T.);
#26769=ADVANCED_FACE('',(#7945),#1460,.T.);
#26770=ADVANCED_FACE('',(#7946),#392,.T.);
#26771=ADVANCED_FACE('',(#7947),#1461,.T.);
#26772=ADVANCED_FACE('',(#7948),#393,.T.);
#26773=ADVANCED_FACE('',(#7949),#6701,.T.);
#26774=ADVANCED_FACE('',(#7950),#1462,.T.);
#26775=ADVANCED_FACE('',(#7951),#6702,.T.);
#26776=ADVANCED_FACE('',(#7952,#709,#710,#711,#712),#1463,.T.);
#26777=ADVANCED_FACE('',(#7953),#1464,.T.);
#26778=ADVANCED_FACE('',(#7954),#394,.T.);
#26779=ADVANCED_FACE('',(#7955),#1465,.T.);
#26780=ADVANCED_FACE('',(#7956),#395,.T.);
#26781=ADVANCED_FACE('',(#7957),#1466,.T.);
#26782=ADVANCED_FACE('',(#7958),#396,.T.);
#26783=ADVANCED_FACE('',(#7959),#1467,.T.);
#26784=ADVANCED_FACE('',(#7960),#397,.T.);
#26785=ADVANCED_FACE('',(#7961),#6703,.T.);
#26786=ADVANCED_FACE('',(#7962),#1468,.T.);
#26787=ADVANCED_FACE('',(#7963),#6704,.T.);
#26788=ADVANCED_FACE('',(#7964),#1469,.T.);
#26789=ADVANCED_FACE('',(#7965),#1470,.F.);
#26790=ADVANCED_FACE('',(#7966),#6705,.T.);
#26791=ADVANCED_FACE('',(#7967),#1471,.T.);
#26792=ADVANCED_FACE('',(#7968),#6706,.T.);
#26793=ADVANCED_FACE('',(#7969),#1472,.T.);
#26794=ADVANCED_FACE('',(#7970),#6707,.F.);
#26795=ADVANCED_FACE('',(#7971),#6708,.F.);
#26796=ADVANCED_FACE('',(#7972),#6709,.F.);
#26797=ADVANCED_FACE('',(#7973),#6710,.F.);
#26798=ADVANCED_FACE('',(#7974),#1473,.T.);
#27235=CLOSED_SHELL('',(#26752,#26753,#26754,#26755,#26756,#26757,#26758,
#26759,#26760,#26761,#26762,#26763,#26764,#26765,#26766,#26767,#26768,#26769,
#26770,#26771,#26772,#26773,#26774,#26775,#26776,#26777,#26778,#26779,#26780,
#26781,#26782,#26783,#26784,#26785,#26786,#26787,#26788,#26789,#26790,#26791,
#26792,#26793,#26794,#26795,#26796,#26797,#26798));
#29306=AXIS2_PLACEMENT_3D('',#45869,#35326,#35327);
#29307=AXIS2_PLACEMENT_3D('',#45870,#35328,#35329);
#29308=AXIS2_PLACEMENT_3D('',#45879,#35334,#35335);
#29309=AXIS2_PLACEMENT_3D('',#45883,#35337,#35338);
#29310=AXIS2_PLACEMENT_3D('',#45884,#35339,#35340);
#29311=AXIS2_PLACEMENT_3D('',#45885,#35341,#35342);
#29312=AXIS2_PLACEMENT_3D('',#45891,#35346,#35347);
#29313=AXIS2_PLACEMENT_3D('',#45895,#35349,#35350);
#29314=AXIS2_PLACEMENT_3D('',#45896,#35351,#35352);
#29315=AXIS2_PLACEMENT_3D('',#45897,#35353,#35354);
#29316=AXIS2_PLACEMENT_3D('',#45903,#35358,#35359);
#29317=AXIS2_PLACEMENT_3D('',#45907,#35361,#35362);
#29318=AXIS2_PLACEMENT_3D('',#45908,#35363,#35364);
#29319=AXIS2_PLACEMENT_3D('',#45909,#35365,#35366);
#29320=AXIS2_PLACEMENT_3D('',#45915,#35370,#35371);
#29321=AXIS2_PLACEMENT_3D('',#45916,#35372,#35373);
#29322=AXIS2_PLACEMENT_3D('',#45917,#35374,#35375);
#29323=AXIS2_PLACEMENT_3D('',#45918,#35376,#35377);
#29324=AXIS2_PLACEMENT_3D('',#45922,#35379,#35380);
#29325=AXIS2_PLACEMENT_3D('',#45924,#35382,#35383);
#29326=AXIS2_PLACEMENT_3D('',#45928,#35386,#35387);
#29327=AXIS2_PLACEMENT_3D('',#45931,#35389,#35390);
#29328=AXIS2_PLACEMENT_3D('',#45932,#35391,#35392);
#29329=AXIS2_PLACEMENT_3D('',#45936,#35395,#35396);
#29330=AXIS2_PLACEMENT_3D('',#45938,#35397,#35398);
#29331=AXIS2_PLACEMENT_3D('',#45940,#35399,#35400);
#29332=AXIS2_PLACEMENT_3D('',#45942,#35401,#35402);
#29333=AXIS2_PLACEMENT_3D('',#45944,#35403,#35404);
#29334=AXIS2_PLACEMENT_3D('',#45949,#35406,#35407);
#29335=AXIS2_PLACEMENT_3D('',#45953,#35409,#35410);
#29336=AXIS2_PLACEMENT_3D('',#45957,#35412,#35413);
#29337=AXIS2_PLACEMENT_3D('',#45960,#35415,#35416);
#29338=AXIS2_PLACEMENT_3D('',#45961,#35417,#35418);
#29339=AXIS2_PLACEMENT_3D('',#45967,#35422,#35423);
#29340=AXIS2_PLACEMENT_3D('',#45971,#35425,#35426);
#29341=AXIS2_PLACEMENT_3D('',#45972,#35427,#35428);
#29342=AXIS2_PLACEMENT_3D('',#45973,#35429,#35430);
#29343=AXIS2_PLACEMENT_3D('',#45979,#35434,#35435);
#29344=AXIS2_PLACEMENT_3D('',#45983,#35437,#35438);
#29345=AXIS2_PLACEMENT_3D('',#45984,#35439,#35440);
#29346=AXIS2_PLACEMENT_3D('',#45985,#35441,#35442);
#29347=AXIS2_PLACEMENT_3D('',#45990,#35446,#35447);
#29348=AXIS2_PLACEMENT_3D('',#45993,#35449,#35450);
#29349=AXIS2_PLACEMENT_3D('',#45994,#35451,#35452);
#29350=AXIS2_PLACEMENT_3D('',#45998,#35455,#35456);
#29351=AXIS2_PLACEMENT_3D('',#45999,#35457,#35458);
#29352=AXIS2_PLACEMENT_3D('',#46000,#35459,#35460);
#29353=AXIS2_PLACEMENT_3D('',#46003,#35463,#35464);
#29354=AXIS2_PLACEMENT_3D('',#46005,#35466,#35467);
#29355=AXIS2_PLACEMENT_3D('',#46006,#35468,#35469);
#29356=AXIS2_PLACEMENT_3D('',#46008,#35470,#35471);
#29357=AXIS2_PLACEMENT_3D('',#46010,#35472,#35473);
#29358=AXIS2_PLACEMENT_3D('',#46012,#35474,#35475);
#29359=AXIS2_PLACEMENT_3D('',#46014,#35476,#35477);
#29360=AXIS2_PLACEMENT_3D('',#46015,#35478,#35479);
#29361=AXIS2_PLACEMENT_3D('',#46024,#35484,#35485);
#29362=AXIS2_PLACEMENT_3D('',#46028,#35487,#35488);
#29363=AXIS2_PLACEMENT_3D('',#46029,#35489,#35490);
#29364=AXIS2_PLACEMENT_3D('',#46030,#35491,#35492);
#29365=AXIS2_PLACEMENT_3D('',#46036,#35496,#35497);
#29366=AXIS2_PLACEMENT_3D('',#46040,#35499,#35500);
#29367=AXIS2_PLACEMENT_3D('',#46041,#35501,#35502);
#29368=AXIS2_PLACEMENT_3D('',#46042,#35503,#35504);
#29369=AXIS2_PLACEMENT_3D('',#46048,#35508,#35509);
#29370=AXIS2_PLACEMENT_3D('',#46052,#35511,#35512);
#29371=AXIS2_PLACEMENT_3D('',#46053,#35513,#35514);
#29372=AXIS2_PLACEMENT_3D('',#46054,#35515,#35516);
#29373=AXIS2_PLACEMENT_3D('',#46060,#35520,#35521);
#29374=AXIS2_PLACEMENT_3D('',#46061,#35522,#35523);
#29375=AXIS2_PLACEMENT_3D('',#46062,#35524,#35525);
#29376=AXIS2_PLACEMENT_3D('',#46063,#35526,#35527);
#29377=AXIS2_PLACEMENT_3D('',#46066,#35530,#35531);
#29378=AXIS2_PLACEMENT_3D('',#46068,#35533,#35534);
#29379=AXIS2_PLACEMENT_3D('',#46070,#35536,#35537);
#29380=AXIS2_PLACEMENT_3D('',#46072,#35539,#35540);
#29381=AXIS2_PLACEMENT_3D('',#46073,#35541,#35542);
#29382=AXIS2_PLACEMENT_3D('',#46075,#35544,#35545);
#29383=AXIS2_PLACEMENT_3D('',#46077,#35547,#35548);
#29384=AXIS2_PLACEMENT_3D('',#46079,#35550,#35551);
#29385=AXIS2_PLACEMENT_3D('',#46080,#35552,#35553);
#29386=AXIS2_PLACEMENT_3D('',#46082,#35555,#35556);
#29387=AXIS2_PLACEMENT_3D('',#46084,#35558,#35559);
#29388=AXIS2_PLACEMENT_3D('',#46086,#35561,#35562);
#29389=AXIS2_PLACEMENT_3D('',#46088,#35564,#35565);
#35326=DIRECTION('axis',(0.,0.,1.));
#35327=DIRECTION('refdir',(1.,0.,0.));
#35328=DIRECTION('center_axis',(-0.707106781186548,0.,-0.707106781186548));
#35329=DIRECTION('ref_axis',(-0.707106781186548,0.,0.707106781186548));
#35330=DIRECTION('',(-0.707106781186532,0.,0.707106781186563));
#35331=DIRECTION('',(0.,1.,0.));
#35332=DIRECTION('',(0.707106781186548,0.,-0.707106781186548));
#35333=DIRECTION('',(0.,-1.,0.));
#35334=DIRECTION('center_axis',(1.,0.,0.));
#35335=DIRECTION('ref_axis',(0.,-1.,-1.77635683940024E-15));
#35336=DIRECTION('',(-0.707106781186548,0.707106781186548,0.));
#35337=DIRECTION('center_axis',(1.,0.,0.));
#35338=DIRECTION('ref_axis',(0.,-1.,-1.77635683940024E-15));
#35339=DIRECTION('center_axis',(-1.,0.,0.));
#35340=DIRECTION('ref_axis',(0.,-1.,-1.77635683940024E-15));
#35341=DIRECTION('center_axis',(-0.707106781186548,-0.707106781186548,0.));
#35342=DIRECTION('ref_axis',(0.,0.,1.));
#35343=DIRECTION('',(-0.707106781186548,0.707106781186548,0.));
#35344=DIRECTION('',(0.,0.,-1.));
#35345=DIRECTION('',(0.,0.,1.));
#35346=DIRECTION('center_axis',(1.,0.,0.));
#35347=DIRECTION('ref_axis',(0.,-3.55271367880049E-15,1.));
#35348=DIRECTION('',(-0.707106781186548,0.,-0.707106781186548));
#35349=DIRECTION('center_axis',(1.,0.,0.));
#35350=DIRECTION('ref_axis',(0.,-3.5527136788005E-15,1.));
#35351=DIRECTION('center_axis',(-1.,0.,0.));
#35352=DIRECTION('ref_axis',(0.,-3.55271367880049E-15,1.));
#35353=DIRECTION('center_axis',(-0.707106781186548,0.,0.707106781186548));
#35354=DIRECTION('ref_axis',(0.707106781186548,0.,0.707106781186548));
#35355=DIRECTION('',(-0.7071067811865,0.,-0.707106781186595));
#35356=DIRECTION('',(0.,-1.,0.));
#35357=DIRECTION('',(0.,1.,0.));
#35358=DIRECTION('center_axis',(1.,0.,0.));
#35359=DIRECTION('ref_axis',(0.,1.,1.77635683940024E-15));
#35360=DIRECTION('',(-0.707106781186548,-0.707106781186548,0.));
#35361=DIRECTION('center_axis',(1.,0.,0.));
#35362=DIRECTION('ref_axis',(0.,1.,1.77635683940024E-15));
#35363=DIRECTION('center_axis',(-1.,0.,0.));
#35364=DIRECTION('ref_axis',(0.,1.,1.77635683940024E-15));
#35365=DIRECTION('center_axis',(-0.707106781186548,0.707106781186548,0.));
#35366=DIRECTION('ref_axis',(0.,0.,1.));
#35367=DIRECTION('',(-0.70710678118661,-0.707106781186485,0.));
#35368=DIRECTION('',(0.,0.,1.));
#35369=DIRECTION('',(0.,0.,-1.));
#35370=DIRECTION('center_axis',(1.,0.,0.));
#35371=DIRECTION('ref_axis',(0.,7.10542735760099E-15,-1.));
#35372=DIRECTION('center_axis',(1.,0.,0.));
#35373=DIRECTION('ref_axis',(0.,7.10542735760099E-15,-1.));
#35374=DIRECTION('center_axis',(-1.,0.,0.));
#35375=DIRECTION('ref_axis',(0.,7.10542735760099E-15,-1.));
#35376=DIRECTION('center_axis',(-1.,0.,0.));
#35377=DIRECTION('ref_axis',(0.,-3.55271367880049E-15,1.));
#35378=DIRECTION('',(-1.,0.,0.));
#35379=DIRECTION('center_axis',(1.,0.,0.));
#35380=DIRECTION('ref_axis',(0.,-3.55271367880049E-15,1.));
#35381=DIRECTION('',(-1.,0.,0.));
#35382=DIRECTION('center_axis',(0.,-1.,0.));
#35383=DIRECTION('ref_axis',(0.,0.,1.));
#35384=DIRECTION('',(-1.,0.,0.));
#35385=DIRECTION('',(0.,0.,-1.));
#35386=DIRECTION('center_axis',(-1.,0.,0.));
#35387=DIRECTION('ref_axis',(0.,-1.,-1.77635683940024E-15));
#35388=DIRECTION('',(-1.,0.,0.));
#35389=DIRECTION('center_axis',(1.,0.,0.));
#35390=DIRECTION('ref_axis',(0.,-1.,-1.77635683940024E-15));
#35391=DIRECTION('center_axis',(0.,0.,-1.));
#35392=DIRECTION('ref_axis',(0.,-1.,0.));
#35393=DIRECTION('',(-1.,0.,0.));
#35394=DIRECTION('',(0.,1.,0.));
#35395=DIRECTION('center_axis',(1.,0.,0.));
#35396=DIRECTION('ref_axis',(0.,0.,-1.));
#35397=DIRECTION('center_axis',(1.,0.,0.));
#35398=DIRECTION('ref_axis',(0.,0.,-1.));
#35399=DIRECTION('center_axis',(1.,0.,0.));
#35400=DIRECTION('ref_axis',(0.,0.,-1.));
#35401=DIRECTION('center_axis',(1.,0.,0.));
#35402=DIRECTION('ref_axis',(0.,0.,-1.));
#35403=DIRECTION('center_axis',(1.,0.,0.));
#35404=DIRECTION('ref_axis',(0.,0.,-1.));
#35405=DIRECTION('',(0.,1.,0.));
#35406=DIRECTION('center_axis',(1.,0.,0.));
#35407=DIRECTION('ref_axis',(0.,0.,-1.));
#35408=DIRECTION('',(0.,0.,1.));
#35409=DIRECTION('center_axis',(1.,0.,0.));
#35410=DIRECTION('ref_axis',(0.,1.,-4.44089209850064E-15));
#35411=DIRECTION('',(0.,-1.,0.));
#35412=DIRECTION('center_axis',(1.,0.,0.));
#35413=DIRECTION('ref_axis',(0.,-4.44089209850061E-15,1.));
#35414=DIRECTION('',(0.,0.,-1.));
#35415=DIRECTION('center_axis',(1.,0.,0.));
#35416=DIRECTION('ref_axis',(0.,-1.,-4.4408920985006E-15));
#35417=DIRECTION('center_axis',(0.707106781186548,0.,-0.707106781186548));
#35418=DIRECTION('ref_axis',(-0.707106781186548,0.,-0.707106781186548));
#35419=DIRECTION('',(0.707106781186548,0.,0.707106781186548));
#35420=DIRECTION('',(0.,-1.,0.));
#35421=DIRECTION('',(-0.707106781186532,0.,-0.707106781186563));
#35422=DIRECTION('center_axis',(-1.,0.,0.));
#35423=DIRECTION('ref_axis',(0.,7.10542735760099E-15,-1.));
#35424=DIRECTION('',(0.707106781186548,-0.707106781186548,0.));
#35425=DIRECTION('center_axis',(-1.,0.,0.));
#35426=DIRECTION('ref_axis',(0.,7.10542735760099E-15,-1.));
#35427=DIRECTION('center_axis',(1.,0.,0.));
#35428=DIRECTION('ref_axis',(0.,7.10542735760099E-15,-1.));
#35429=DIRECTION('center_axis',(0.707106781186548,0.707106781186548,0.));
#35430=DIRECTION('ref_axis',(0.,0.,-1.));
#35431=DIRECTION('',(0.707106781186548,-0.707106781186548,0.));
#35432=DIRECTION('',(0.,0.,-1.));
#35433=DIRECTION('',(0.,0.,1.));
#35434=DIRECTION('center_axis',(-1.,0.,0.));
#35435=DIRECTION('ref_axis',(0.,1.,1.77635683940024E-15));
#35436=DIRECTION('',(0.707106781186516,0.,-0.707106781186579));
#35437=DIRECTION('center_axis',(-1.,0.,0.));
#35438=DIRECTION('ref_axis',(0.,1.,1.77635683940024E-15));
#35439=DIRECTION('center_axis',(1.,0.,0.));
#35440=DIRECTION('ref_axis',(0.,1.,1.77635683940024E-15));
#35441=DIRECTION('center_axis',(0.707106781186548,0.,0.707106781186548));
#35442=DIRECTION('ref_axis',(0.707106781186548,0.,-0.707106781186548));
#35443=DIRECTION('',(0.707106781186548,0.,-0.707106781186548));
#35444=DIRECTION('',(0.,1.,0.));
#35445=DIRECTION('',(0.,-1.,0.));
#35446=DIRECTION('center_axis',(-1.,0.,0.));
#35447=DIRECTION('ref_axis',(0.,-3.55271367880049E-15,1.));
#35448=DIRECTION('',(0.707106781186548,0.707106781186548,0.));
#35449=DIRECTION('center_axis',(-1.,0.,0.));
#35450=DIRECTION('ref_axis',(0.,-3.5527136788005E-15,1.));
#35451=DIRECTION('center_axis',(0.707106781186548,-0.707106781186548,0.));
#35452=DIRECTION('ref_axis',(0.,0.,-1.));
#35453=DIRECTION('',(0.707106781186548,0.707106781186548,0.));
#35454=DIRECTION('',(0.,0.,1.));
#35455=DIRECTION('center_axis',(-1.,0.,0.));
#35456=DIRECTION('ref_axis',(0.,-1.,-1.77635683940024E-15));
#35457=DIRECTION('center_axis',(-1.,0.,0.));
#35458=DIRECTION('ref_axis',(0.,-1.,-1.77635683940024E-15));
#35459=DIRECTION('center_axis',(-1.,0.,0.));
#35460=DIRECTION('ref_axis',(0.,1.,1.77635683940024E-15));
#35461=DIRECTION('',(-1.,0.,0.));
#35462=DIRECTION('',(-1.,0.,0.));
#35463=DIRECTION('center_axis',(0.,1.,0.));
#35464=DIRECTION('ref_axis',(0.,0.,-1.));
#35465=DIRECTION('',(-1.,0.,0.));
#35466=DIRECTION('center_axis',(-1.,0.,0.));
#35467=DIRECTION('ref_axis',(0.,7.10542735760099E-15,-1.));
#35468=DIRECTION('center_axis',(1.,0.,0.));
#35469=DIRECTION('ref_axis',(0.,0.,-1.));
#35470=DIRECTION('center_axis',(-1.,0.,0.));
#35471=DIRECTION('ref_axis',(0.,0.,-1.));
#35472=DIRECTION('center_axis',(-1.,0.,0.));
#35473=DIRECTION('ref_axis',(0.,0.,-1.));
#35474=DIRECTION('center_axis',(-1.,0.,0.));
#35475=DIRECTION('ref_axis',(0.,0.,-1.));
#35476=DIRECTION('center_axis',(-1.,0.,0.));
#35477=DIRECTION('ref_axis',(0.,0.,-1.));
#35478=DIRECTION('center_axis',(-0.70710678118654,0.,-0.707106781186555));
#35479=DIRECTION('ref_axis',(-0.707106781186555,0.,0.70710678118654));
#35480=DIRECTION('',(-0.707106781186548,0.,0.707106781186548));
#35481=DIRECTION('',(0.,1.,0.));
#35482=DIRECTION('',(0.707106781186555,0.,-0.70710678118654));
#35483=DIRECTION('',(0.,-1.,0.));
#35484=DIRECTION('center_axis',(1.,0.,0.));
#35485=DIRECTION('ref_axis',(0.,-1.,-4.4408920985006E-15));
#35486=DIRECTION('',(-0.707106781186548,0.707106781186548,0.));
#35487=DIRECTION('center_axis',(1.,0.,0.));
#35488=DIRECTION('ref_axis',(0.,-1.,-4.4408920985006E-15));
#35489=DIRECTION('center_axis',(-1.,0.,0.));
#35490=DIRECTION('ref_axis',(0.,-1.,-4.4408920985006E-15));
#35491=DIRECTION('center_axis',(-0.707106781186532,-0.707106781186563,0.));
#35492=DIRECTION('ref_axis',(0.,0.,1.));
#35493=DIRECTION('',(-0.707106781186563,0.707106781186532,1.57009245868377E-14));
#35494=DIRECTION('',(0.,0.,-1.));
#35495=DIRECTION('',(0.,0.,1.));
#35496=DIRECTION('center_axis',(1.,0.,0.));
#35497=DIRECTION('ref_axis',(0.,-4.44089209850061E-15,1.));
#35498=DIRECTION('',(-0.707106781186548,0.,-0.707106781186548));
#35499=DIRECTION('center_axis',(1.,0.,0.));
#35500=DIRECTION('ref_axis',(0.,-4.44089209850061E-15,1.));
#35501=DIRECTION('center_axis',(-1.,0.,0.));
#35502=DIRECTION('ref_axis',(0.,-4.44089209850061E-15,1.));
#35503=DIRECTION('center_axis',(-0.70710678118654,0.,0.707106781186555));
#35504=DIRECTION('ref_axis',(0.707106781186555,0.,0.70710678118654));
#35505=DIRECTION('',(-0.707106781186548,0.,-0.707106781186548));
#35506=DIRECTION('',(0.,-1.,0.));
#35507=DIRECTION('',(0.,1.,0.));
#35508=DIRECTION('center_axis',(1.,0.,0.));
#35509=DIRECTION('ref_axis',(0.,1.,-4.44089209850064E-15));
#35510=DIRECTION('',(-0.707106781186548,-0.707106781186548,0.));
#35511=DIRECTION('center_axis',(1.,0.,0.));
#35512=DIRECTION('ref_axis',(0.,1.,-4.44089209850064E-15));
#35513=DIRECTION('center_axis',(-1.,0.,0.));
#35514=DIRECTION('ref_axis',(0.,1.,-4.44089209850064E-15));
#35515=DIRECTION('center_axis',(-0.707106781186532,0.707106781186563,0.));
#35516=DIRECTION('ref_axis',(0.,0.,1.));
#35517=DIRECTION('',(-0.707106781186563,-0.707106781186532,-1.57009245868377E-14));
#35518=DIRECTION('',(0.,0.,1.));
#35519=DIRECTION('',(0.,0.,-1.));
#35520=DIRECTION('center_axis',(1.,0.,0.));
#35521=DIRECTION('ref_axis',(0.,0.,-1.));
#35522=DIRECTION('center_axis',(1.,0.,0.));
#35523=DIRECTION('ref_axis',(0.,0.,-1.));
#35524=DIRECTION('center_axis',(-1.,0.,0.));
#35525=DIRECTION('ref_axis',(0.,0.,-1.));
#35526=DIRECTION('center_axis',(-1.,0.,0.));
#35527=DIRECTION('ref_axis',(0.,-4.44089209850061E-15,1.));
#35528=DIRECTION('',(-1.,0.,0.));
#35529=DIRECTION('',(-1.,0.,0.));
#35530=DIRECTION('center_axis',(0.,-1.,0.));
#35531=DIRECTION('ref_axis',(0.,0.,1.));
#35532=DIRECTION('',(-1.,0.,0.));
#35533=DIRECTION('center_axis',(-1.,0.,0.));
#35534=DIRECTION('ref_axis',(0.,-1.,-4.4408920985006E-15));
#35535=DIRECTION('',(-1.,0.,0.));
#35536=DIRECTION('center_axis',(0.,0.,-1.));
#35537=DIRECTION('ref_axis',(0.,-1.,0.));
#35538=DIRECTION('',(-1.,0.,0.));
#35539=DIRECTION('center_axis',(1.,0.,0.));
#35540=DIRECTION('ref_axis',(0.,0.,-1.));
#35541=DIRECTION('center_axis',(-1.,0.,0.));
#35542=DIRECTION('ref_axis',(0.,0.,-1.));
#35543=DIRECTION('',(-1.,0.,0.));
#35544=DIRECTION('center_axis',(0.,1.,0.));
#35545=DIRECTION('ref_axis',(0.,0.,-1.));
#35546=DIRECTION('',(-1.,0.,0.));
#35547=DIRECTION('center_axis',(-1.,0.,0.));
#35548=DIRECTION('ref_axis',(0.,1.,-4.44089209850064E-15));
#35549=DIRECTION('',(-1.,0.,0.));
#35550=DIRECTION('center_axis',(0.,0.,1.));
#35551=DIRECTION('ref_axis',(0.,1.,0.));
#35552=DIRECTION('center_axis',(-1.,0.,0.));
#35553=DIRECTION('ref_axis',(0.,0.,-1.));
#35554=DIRECTION('',(-1.,0.,0.));
#35555=DIRECTION('center_axis',(-1.,0.,0.));
#35556=DIRECTION('ref_axis',(0.,0.,-1.));
#35557=DIRECTION('',(-1.,0.,0.));
#35558=DIRECTION('center_axis',(-1.,0.,0.));
#35559=DIRECTION('ref_axis',(0.,0.,-1.));
#35560=DIRECTION('',(-1.,0.,0.));
#35561=DIRECTION('center_axis',(-1.,0.,0.));
#35562=DIRECTION('ref_axis',(0.,0.,-1.));
#35563=DIRECTION('',(-1.,0.,0.));
#35564=DIRECTION('center_axis',(0.,0.,1.));
#35565=DIRECTION('ref_axis',(0.,1.,0.));
#45869=CARTESIAN_POINT('',(0.,0.,0.));
#45870=CARTESIAN_POINT('Origin',(-56.4,179.5,-41.9));
#45871=CARTESIAN_POINT('',(-56.3,142.,-42.));
#45872=CARTESIAN_POINT('',(-56.5,142.,-41.8));
#45873=CARTESIAN_POINT('',(-56.3,142.,-42.));
#45874=CARTESIAN_POINT('',(-56.5,192.,-41.8));
#45875=CARTESIAN_POINT('',(-56.5,179.5,-41.8));
#45876=CARTESIAN_POINT('',(-56.3,192.,-42.));
#45877=CARTESIAN_POINT('',(-56.5,192.,-41.8));
#45878=CARTESIAN_POINT('',(-56.3,179.5,-42.));
#45879=CARTESIAN_POINT('Origin',(-56.4,142.,-37.));
#45880=CARTESIAN_POINT('',(-56.3,137.,-37.));
#45881=CARTESIAN_POINT('',(-56.5,137.2,-37.));
#45882=CARTESIAN_POINT('',(-56.3,137.,-37.));
#45883=CARTESIAN_POINT('Origin',(-56.5,142.,-37.));
#45884=CARTESIAN_POINT('Origin',(-56.3,142.,-37.));
#45885=CARTESIAN_POINT('Origin',(-56.4,137.1,-18.5));
#45886=CARTESIAN_POINT('',(-56.3,137.,37.));
#45887=CARTESIAN_POINT('',(-56.5,137.2,37.));
#45888=CARTESIAN_POINT('',(-56.3,137.,37.));
#45889=CARTESIAN_POINT('',(-56.5,137.2,-18.5));
#45890=CARTESIAN_POINT('',(-56.3,137.,-18.5));
#45891=CARTESIAN_POINT('Origin',(-56.4,142.,37.));
#45892=CARTESIAN_POINT('',(-56.3,142.,42.));
#45893=CARTESIAN_POINT('',(-56.5,142.,41.8));
#45894=CARTESIAN_POINT('',(-56.3,142.,42.));
#45895=CARTESIAN_POINT('Origin',(-56.5,142.,37.));
#45896=CARTESIAN_POINT('Origin',(-56.3,142.,37.));
#45897=CARTESIAN_POINT('Origin',(-56.4,154.5,41.9));
#45898=CARTESIAN_POINT('',(-56.3,192.,42.));
#45899=CARTESIAN_POINT('',(-56.5,192.,41.8));
#45900=CARTESIAN_POINT('',(-56.3,192.,42.));
#45901=CARTESIAN_POINT('',(-56.5,154.5,41.8));
#45902=CARTESIAN_POINT('',(-56.3,154.5,42.));
#45903=CARTESIAN_POINT('Origin',(-56.4,192.,37.));
#45904=CARTESIAN_POINT('',(-56.3,197.,37.));
#45905=CARTESIAN_POINT('',(-56.5,196.8,37.));
#45906=CARTESIAN_POINT('',(-56.3,197.,37.));
#45907=CARTESIAN_POINT('Origin',(-56.5,192.,37.));
#45908=CARTESIAN_POINT('Origin',(-56.3,192.,37.));
#45909=CARTESIAN_POINT('Origin',(-56.4,196.9,18.5));
#45910=CARTESIAN_POINT('',(-56.3,197.,-37.));
#45911=CARTESIAN_POINT('',(-56.5,196.8,-37.));
#45912=CARTESIAN_POINT('',(-56.3,197.,-37.));
#45913=CARTESIAN_POINT('',(-56.5,196.8,18.5));
#45914=CARTESIAN_POINT('',(-56.3,197.,18.5));
#45915=CARTESIAN_POINT('Origin',(-56.4,192.,-37.));
#45916=CARTESIAN_POINT('Origin',(-56.5,192.,-37.));
#45917=CARTESIAN_POINT('Origin',(-56.3,192.,-37.));
#45918=CARTESIAN_POINT('Origin',(-55.,142.,37.));
#45919=CARTESIAN_POINT('',(-55.2,137.,37.));
#45920=CARTESIAN_POINT('',(-55.,137.,37.));
#45921=CARTESIAN_POINT('',(-55.2,142.,42.));
#45922=CARTESIAN_POINT('Origin',(-55.2,142.,37.));
#45923=CARTESIAN_POINT('',(-55.,142.,42.));
#45924=CARTESIAN_POINT('Origin',(-55.,137.,-37.));
#45925=CARTESIAN_POINT('',(-55.2,137.,-37.));
#45926=CARTESIAN_POINT('',(-55.,137.,-37.));
#45927=CARTESIAN_POINT('',(-55.2,137.,-18.5));
#45928=CARTESIAN_POINT('Origin',(-55.,142.,-37.));
#45929=CARTESIAN_POINT('',(-55.2,142.,-42.));
#45930=CARTESIAN_POINT('',(-55.,142.,-42.));
#45931=CARTESIAN_POINT('Origin',(-55.2,142.,-37.));
#45932=CARTESIAN_POINT('Origin',(-55.,192.,-42.));
#45933=CARTESIAN_POINT('',(-55.2,192.,-42.));
#45934=CARTESIAN_POINT('',(-55.,192.,-42.));
#45935=CARTESIAN_POINT('',(-55.2,179.5,-42.));
#45936=CARTESIAN_POINT('Origin',(-56.5,167.,8.88178419700125E-15));
#45937=CARTESIAN_POINT('',(-56.5,193.,40.75));
#45938=CARTESIAN_POINT('Origin',(-56.5,193.,38.));
#45939=CARTESIAN_POINT('',(-56.5,141.,-35.25));
#45940=CARTESIAN_POINT('Origin',(-56.5,141.,-38.));
#45941=CARTESIAN_POINT('',(-56.5,141.,40.75));
#45942=CARTESIAN_POINT('Origin',(-56.5,141.,38.));
#45943=CARTESIAN_POINT('',(-56.5,193.,-35.25));
#45944=CARTESIAN_POINT('Origin',(-56.5,193.,-38.));
#45945=CARTESIAN_POINT('',(-56.5,151.,-30.));
#45946=CARTESIAN_POINT('',(-56.5,183.,-30.));
#45947=CARTESIAN_POINT('',(-56.5,175.,-30.));
#45948=CARTESIAN_POINT('',(-56.5,187.,-26.));
#45949=CARTESIAN_POINT('Origin',(-56.5,183.,-26.));
#45950=CARTESIAN_POINT('',(-56.5,187.,26.));
#45951=CARTESIAN_POINT('',(-56.5,187.,13.));
#45952=CARTESIAN_POINT('',(-56.5,183.,30.));
#45953=CARTESIAN_POINT('Origin',(-56.5,183.,26.));
#45954=CARTESIAN_POINT('',(-56.5,151.,30.));
#45955=CARTESIAN_POINT('',(-56.5,159.,30.));
#45956=CARTESIAN_POINT('',(-56.5,147.,26.));
#45957=CARTESIAN_POINT('Origin',(-56.5,151.,26.));
#45958=CARTESIAN_POINT('',(-56.5,147.,-26.));
#45959=CARTESIAN_POINT('',(-56.5,147.,-13.));
#45960=CARTESIAN_POINT('Origin',(-56.5,151.,-26.));
#45961=CARTESIAN_POINT('Origin',(-55.1,179.5,-41.9));
#45962=CARTESIAN_POINT('',(-55.,192.,-41.8));
#45963=CARTESIAN_POINT('',(-55.2,192.,-42.));
#45964=CARTESIAN_POINT('',(-55.,142.,-41.8));
#45965=CARTESIAN_POINT('',(-55.,179.5,-41.8));
#45966=CARTESIAN_POINT('',(-55.,142.,-41.8));
#45967=CARTESIAN_POINT('Origin',(-55.1,192.,-37.));
#45968=CARTESIAN_POINT('',(-55.2,197.,-37.));
#45969=CARTESIAN_POINT('',(-55.,196.8,-37.));
#45970=CARTESIAN_POINT('',(-55.2,197.,-37.));
#45971=CARTESIAN_POINT('Origin',(-55.,192.,-37.));
#45972=CARTESIAN_POINT('Origin',(-55.2,192.,-37.));
#45973=CARTESIAN_POINT('Origin',(-55.1,196.9,18.5));
#45974=CARTESIAN_POINT('',(-55.2,197.,37.));
#45975=CARTESIAN_POINT('',(-55.,196.8,37.));
#45976=CARTESIAN_POINT('',(-55.2,197.,37.));
#45977=CARTESIAN_POINT('',(-55.,196.8,18.5));
#45978=CARTESIAN_POINT('',(-55.2,197.,18.5));
#45979=CARTESIAN_POINT('Origin',(-55.1,192.,37.));
#45980=CARTESIAN_POINT('',(-55.2,192.,42.));
#45981=CARTESIAN_POINT('',(-55.,192.,41.8));
#45982=CARTESIAN_POINT('',(-55.2,192.,42.));
#45983=CARTESIAN_POINT('Origin',(-55.,192.,37.));
#45984=CARTESIAN_POINT('Origin',(-55.2,192.,37.));
#45985=CARTESIAN_POINT('Origin',(-55.1,154.5,41.9));
#45986=CARTESIAN_POINT('',(-55.,142.,41.8));
#45987=CARTESIAN_POINT('',(-55.2,142.,42.));
#45988=CARTESIAN_POINT('',(-55.,154.5,41.8));
#45989=CARTESIAN_POINT('',(-55.2,154.5,42.));
#45990=CARTESIAN_POINT('Origin',(-55.1,142.,37.));
#45991=CARTESIAN_POINT('',(-55.,137.2,37.));
#45992=CARTESIAN_POINT('',(-55.2,137.,37.));
#45993=CARTESIAN_POINT('Origin',(-55.,142.,37.));
#45994=CARTESIAN_POINT('Origin',(-55.1,137.1,-18.5));
#45995=CARTESIAN_POINT('',(-55.,137.2,-37.));
#45996=CARTESIAN_POINT('',(-55.2,137.,-37.));
#45997=CARTESIAN_POINT('',(-55.,137.2,-18.5));
#45998=CARTESIAN_POINT('Origin',(-55.1,142.,-37.));
#45999=CARTESIAN_POINT('Origin',(-55.,142.,-37.));
#46000=CARTESIAN_POINT('Origin',(-55.,192.,37.));
#46001=CARTESIAN_POINT('',(-55.,192.,42.));
#46002=CARTESIAN_POINT('',(-55.,197.,37.));
#46003=CARTESIAN_POINT('Origin',(-55.,197.,37.));
#46004=CARTESIAN_POINT('',(-55.,197.,-37.));
#46005=CARTESIAN_POINT('Origin',(-55.,192.,-37.));
#46006=CARTESIAN_POINT('Origin',(-55.,167.,8.88178419700125E-15));
#46007=CARTESIAN_POINT('',(-55.,193.,40.75));
#46008=CARTESIAN_POINT('Origin',(-55.,193.,38.));
#46009=CARTESIAN_POINT('',(-55.,141.,-35.25));
#46010=CARTESIAN_POINT('Origin',(-55.,141.,-38.));
#46011=CARTESIAN_POINT('',(-55.,141.,40.75));
#46012=CARTESIAN_POINT('Origin',(-55.,141.,38.));
#46013=CARTESIAN_POINT('',(-55.,193.,-35.25));
#46014=CARTESIAN_POINT('Origin',(-55.,193.,-38.));
#46015=CARTESIAN_POINT('Origin',(-57.,175.,-29.9));
#46016=CARTESIAN_POINT('',(-56.9,151.,-30.));
#46017=CARTESIAN_POINT('',(-57.1,151.,-29.8));
#46018=CARTESIAN_POINT('',(-56.9,151.,-30.));
#46019=CARTESIAN_POINT('',(-57.1,183.,-29.8));
#46020=CARTESIAN_POINT('',(-57.1,175.,-29.8));
#46021=CARTESIAN_POINT('',(-56.9,183.,-30.));
#46022=CARTESIAN_POINT('',(-57.1,183.,-29.8));
#46023=CARTESIAN_POINT('',(-56.9,175.,-30.));
#46024=CARTESIAN_POINT('Origin',(-57.,151.,-26.));
#46025=CARTESIAN_POINT('',(-56.9,147.,-26.));
#46026=CARTESIAN_POINT('',(-57.1,147.2,-26.));
#46027=CARTESIAN_POINT('',(-56.9,147.,-26.));
#46028=CARTESIAN_POINT('Origin',(-57.1,151.,-26.));
#46029=CARTESIAN_POINT('Origin',(-56.9,151.,-26.));
#46030=CARTESIAN_POINT('Origin',(-57.,147.1,-13.));
#46031=CARTESIAN_POINT('',(-56.9,147.,26.));
#46032=CARTESIAN_POINT('',(-57.1,147.2,26.));
#46033=CARTESIAN_POINT('',(-56.9,147.,26.));
#46034=CARTESIAN_POINT('',(-57.1,147.2,-13.));
#46035=CARTESIAN_POINT('',(-56.9,147.,-13.));
#46036=CARTESIAN_POINT('Origin',(-57.,151.,26.));
#46037=CARTESIAN_POINT('',(-56.9,151.,30.));
#46038=CARTESIAN_POINT('',(-57.1,151.,29.8));
#46039=CARTESIAN_POINT('',(-56.9,151.,30.));
#46040=CARTESIAN_POINT('Origin',(-57.1,151.,26.));
#46041=CARTESIAN_POINT('Origin',(-56.9,151.,26.));
#46042=CARTESIAN_POINT('Origin',(-57.,159.,29.9));
#46043=CARTESIAN_POINT('',(-56.9,183.,30.));
#46044=CARTESIAN_POINT('',(-57.1,183.,29.8));
#46045=CARTESIAN_POINT('',(-56.9,183.,30.));
#46046=CARTESIAN_POINT('',(-57.1,159.,29.8));
#46047=CARTESIAN_POINT('',(-56.9,159.,30.));
#46048=CARTESIAN_POINT('Origin',(-57.,183.,26.));
#46049=CARTESIAN_POINT('',(-56.9,187.,26.));
#46050=CARTESIAN_POINT('',(-57.1,186.8,26.));
#46051=CARTESIAN_POINT('',(-56.9,187.,26.));
#46052=CARTESIAN_POINT('Origin',(-57.1,183.,26.));
#46053=CARTESIAN_POINT('Origin',(-56.9,183.,26.));
#46054=CARTESIAN_POINT('Origin',(-57.,186.9,13.));
#46055=CARTESIAN_POINT('',(-56.9,187.,-26.));
#46056=CARTESIAN_POINT('',(-57.1,186.8,-26.));
#46057=CARTESIAN_POINT('',(-56.9,187.,-26.));
#46058=CARTESIAN_POINT('',(-57.1,186.8,13.));
#46059=CARTESIAN_POINT('',(-56.9,187.,13.));
#46060=CARTESIAN_POINT('Origin',(-57.,183.,-26.));
#46061=CARTESIAN_POINT('Origin',(-57.1,183.,-26.));
#46062=CARTESIAN_POINT('Origin',(-56.9,183.,-26.));
#46063=CARTESIAN_POINT('Origin',(-56.5,151.,26.));
#46064=CARTESIAN_POINT('',(-56.5,147.,26.));
#46065=CARTESIAN_POINT('',(-56.5,151.,30.));
#46066=CARTESIAN_POINT('Origin',(-56.5,147.,-26.));
#46067=CARTESIAN_POINT('',(-56.5,147.,-26.));
#46068=CARTESIAN_POINT('Origin',(-56.5,151.,-26.));
#46069=CARTESIAN_POINT('',(-56.5,151.,-30.));
#46070=CARTESIAN_POINT('Origin',(-56.5,183.,-30.));
#46071=CARTESIAN_POINT('',(-56.5,183.,-30.));
#46072=CARTESIAN_POINT('Origin',(-57.1,167.,0.));
#46073=CARTESIAN_POINT('Origin',(-56.5,183.,-26.));
#46074=CARTESIAN_POINT('',(-56.5,187.,-26.));
#46075=CARTESIAN_POINT('Origin',(-56.5,187.,26.));
#46076=CARTESIAN_POINT('',(-56.5,187.,26.));
#46077=CARTESIAN_POINT('Origin',(-56.5,183.,26.));
#46078=CARTESIAN_POINT('',(-56.5,183.,30.));
#46079=CARTESIAN_POINT('Origin',(-56.5,151.,30.));
#46080=CARTESIAN_POINT('Origin',(-55.,193.,-38.));
#46081=CARTESIAN_POINT('',(-55.,193.,-35.25));
#46082=CARTESIAN_POINT('Origin',(-55.,141.,38.));
#46083=CARTESIAN_POINT('',(-55.,141.,40.75));
#46084=CARTESIAN_POINT('Origin',(-55.,141.,-38.));
#46085=CARTESIAN_POINT('',(-55.,141.,-35.25));
#46086=CARTESIAN_POINT('Origin',(-55.,193.,38.));
#46087=CARTESIAN_POINT('',(-55.,193.,40.75));
#46088=CARTESIAN_POINT('Origin',(-55.,142.,42.));
#55709=UNCERTAINTY_MEASURE_WITH_UNIT(LENGTH_MEASURE(0.01),#55738,
'DISTANCE_ACCURACY_VALUE',
'Maximum model space distance between geometric entities at asserted c
onnectivities');
#55715=UNCERTAINTY_MEASURE_WITH_UNIT(LENGTH_MEASURE(0.01),#55738,
'DISTANCE_ACCURACY_VALUE',
'Maximum model space distance between geometric entities at asserted c
onnectivities');
#55731=(
GEOMETRIC_REPRESENTATION_CONTEXT(3)
GLOBAL_UNCERTAINTY_ASSIGNED_CONTEXT((#55709))
GLOBAL_UNIT_ASSIGNED_CONTEXT((#55738,#55740,#55741))
REPRESENTATION_CONTEXT('','3D')
);
#55737=(
GEOMETRIC_REPRESENTATION_CONTEXT(3)
GLOBAL_UNCERTAINTY_ASSIGNED_CONTEXT((#55715))
GLOBAL_UNIT_ASSIGNED_CONTEXT((#55738,#55740,#55741))
REPRESENTATION_CONTEXT('','3D')
);
#55738=(
LENGTH_UNIT()
NAMED_UNIT(*)
SI_UNIT(.MILLI.,.METRE.)
);
#55740=(
NAMED_UNIT(*)
PLANE_ANGLE_UNIT()
SI_UNIT($,.RADIAN.)
);
#55741=(
NAMED_UNIT(*)
SI_UNIT($,.STERADIAN.)
SOLID_ANGLE_UNIT()
);
#55757=SHAPE_DEFINITION_REPRESENTATION(#55778,#55835);
#55778=PRODUCT_DEFINITION_SHAPE('',$,#55857);
#55835=SHAPE_REPRESENTATION('',(#29306),#55731);
#55841=PRODUCT_DEFINITION_CONTEXT('part definition',#55906,'design');
#55857=PRODUCT_DEFINITION('2026-10-26-00-34-36-690',
'18_Coupling_Window_Plate',#55878,#55841);
#55878=PRODUCT_DEFINITION_FORMATION('',$,#55923);
#55906=APPLICATION_CONTEXT(
'Core Data for Automotive Mechanical Design Process');
#55907=PRODUCT_CONTEXT('part definition',#55906,'mechanical');
#55923=PRODUCT('2026-10-26-00-34-36-690','18_Coupling_Window_Plate',$,(#55907));
#55971=COLOUR_RGB('Light Blue',0.38,0.62,0.78);
#55972=FILL_AREA_STYLE_COLOUR('',#55971);
#55973=FILL_AREA_STYLE('',(#55972));
#55974=SURFACE_STYLE_FILL_AREA(#55973);
#55975=SURFACE_SIDE_STYLE('',(#55974));
#55976=SURFACE_STYLE_USAGE(.BOTH.,#55975);
#55977=PRESENTATION_STYLE_ASSIGNMENT((#55976));
ENDSEC;
END-ISO-10303-21;
